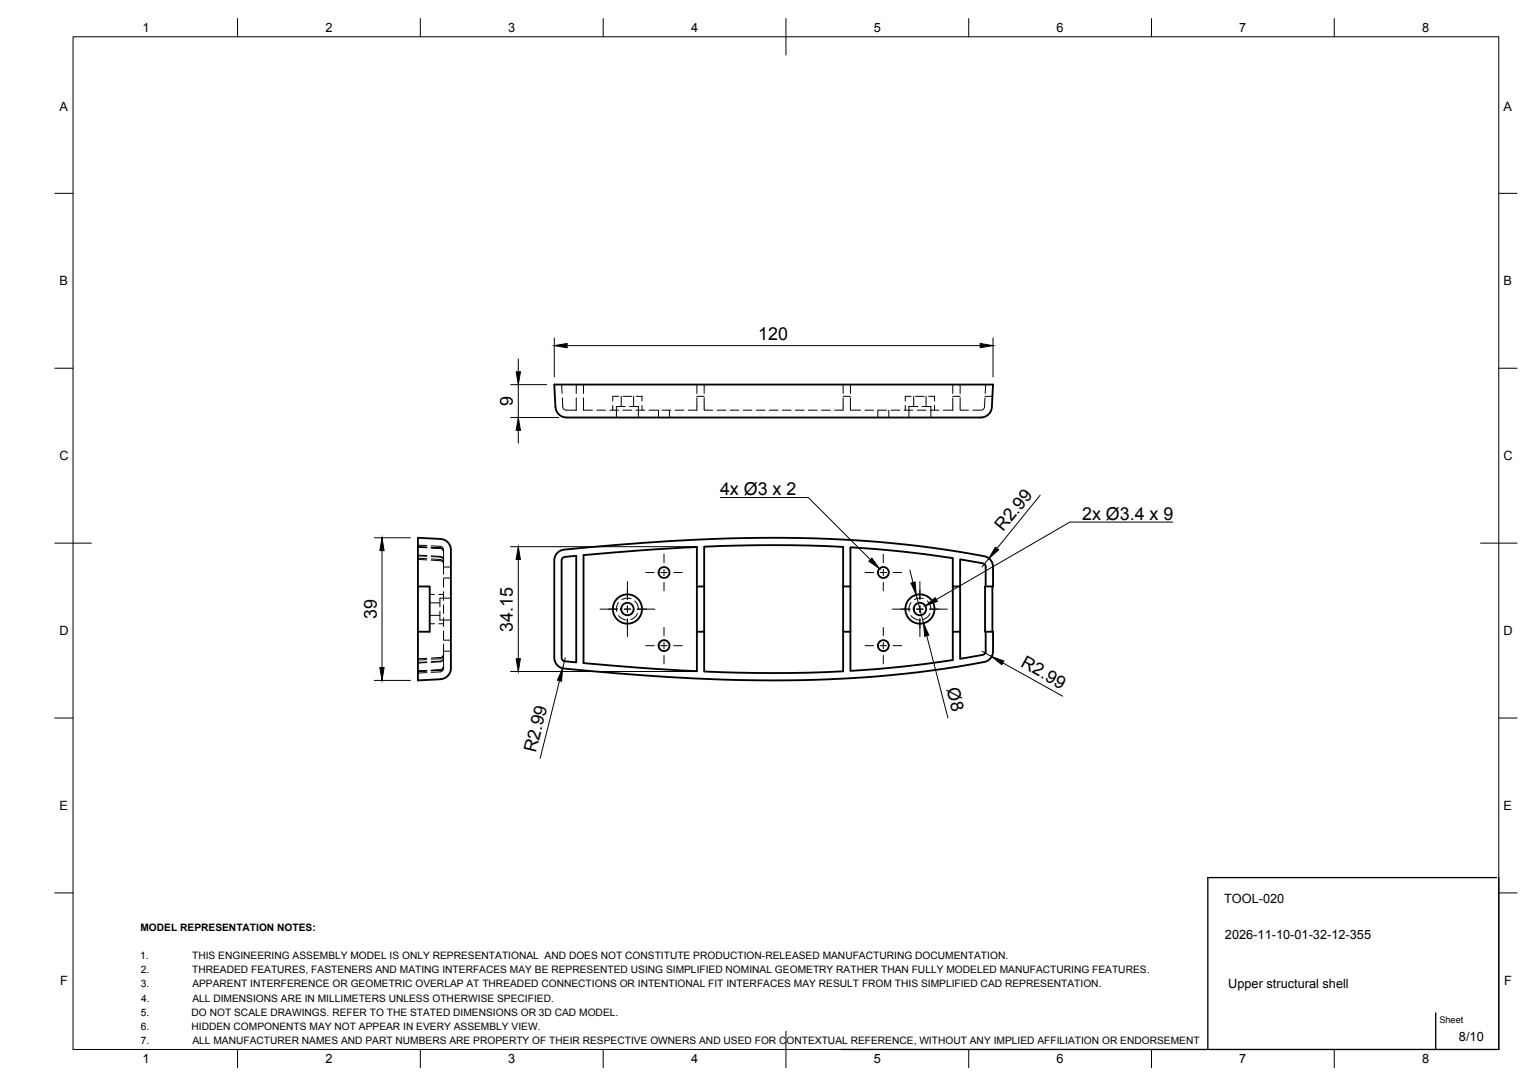
ISO-10303-21;
HEADER;
/* Generated by software containing ST-Developer
 * from STEP Tools, Inc. (www.steptools.com) 
 */

FILE_DESCRIPTION(
/* description */ (''),
/* implementation_level */ '2;1');

FILE_NAME(
/* name */ 'Upper structural shell.step',
/* time_stamp */ '2026-11-10T09:09:39-08:00',
/* author */ (''),
/* organization */ (''),
/* preprocessor_version */ 'ST-DEVELOPER v20.2',
/* originating_system */ 'Autodesk Translation Framework v15.17.0.0',
/* authorisation */ '');

FILE_SCHEMA (('AUTOMOTIVE_DESIGN { 1 0 10303 214 3 1 1 }'));
ENDSEC;

DATA;
#10=MECHANICAL_DESIGN_GEOMETRIC_PRESENTATION_REPRESENTATION('',(#558),#18353);
#75=SPHERICAL_SURFACE('',#6751,0.0999999999999999);
#76=SPHERICAL_SURFACE('',#6754,0.100000000000002);
#77=SPHERICAL_SURFACE('',#6758,0.0999999999999991);
#78=SPHERICAL_SURFACE('',#6762,0.1);
#79=SPHERICAL_SURFACE('',#6767,0.3);
#80=SPHERICAL_SURFACE('',#6771,0.300000000000002);
#81=SPHERICAL_SURFACE('',#6775,0.299999999999999);
#82=SPHERICAL_SURFACE('',#6780,0.3);
#91=B_SPLINE_SURFACE_WITH_KNOTS('',3,3,((#9570,#9571,#9572,#9573),(#9574,
#9575,#9576,#9577),(#9578,#9579,#9580,#9581),(#9582,#9583,#9584,#9585)),
 .UNSPECIFIED.,.F.,.F.,.F.,(4,4),(4,4),(0.0627625298587661,0.3242096015809),
(0.0118073085896899,0.685451490706028),.UNSPECIFIED.);
#92=B_SPLINE_SURFACE_WITH_KNOTS('',3,3,((#9590,#9591,#9592,#9593),(#9594,
#9595,#9596,#9597),(#9598,#9599,#9600,#9601),(#9602,#9603,#9604,#9605)),
 .UNSPECIFIED.,.F.,.F.,.F.,(4,4),(4,4),(0.0225360950145449,0.0483865590996774),
(0.0125659096559557,0.685650832343257),.UNSPECIFIED.);
#93=B_SPLINE_SURFACE_WITH_KNOTS('',3,3,((#9615,#9616,#9617,#9618),(#9619,
#9620,#9621,#9622),(#9623,#9624,#9625,#9626),(#9627,#9628,#9629,#9630),
(#9631,#9632,#9633,#9634)),.UNSPECIFIED.,.F.,.F.,.F.,(4,1,4),(4,4),(0.,
0.571428571428571,1.),(0.74118252158834,3.85438678954986),.UNSPECIFIED.);
#94=B_SPLINE_SURFACE_WITH_KNOTS('',3,3,((#9639,#9640,#9641,#9642),(#9643,
#9644,#9645,#9646),(#9647,#9648,#9649,#9650),(#9651,#9652,#9653,#9654),
(#9655,#9656,#9657,#9658)),.UNSPECIFIED.,.F.,.F.,.F.,(4,1,4),(4,4),(0.,
0.571428571428571,1.),(0.270878787657975,0.54981857912664),
 .UNSPECIFIED.);
#95=B_SPLINE_SURFACE_WITH_KNOTS('',3,3,((#9677,#9678,#9679,#9680),(#9681,
#9682,#9683,#9684),(#9685,#9686,#9687,#9688),(#9689,#9690,#9691,#9692),
(#9693,#9694,#9695,#9696)),.UNSPECIFIED.,.F.,.F.,.F.,(4,1,4),(4,4),(0.,
0.571428571428571,1.),(8.03948512627517,11.1526893942367),.UNSPECIFIED.);
#96=B_SPLINE_SURFACE_WITH_KNOTS('',3,3,((#9701,#9702,#9703,#9704),(#9705,
#9706,#9707,#9708),(#9709,#9710,#9711,#9712),(#9713,#9714,#9715,#9716)),
 .UNSPECIFIED.,.F.,.F.,.F.,(4,4),(4,4),(0.675790398419059,0.937237470141233),
(0.0118073085603101,0.685451490706029),.UNSPECIFIED.);
#97=B_SPLINE_SURFACE_WITH_KNOTS('',3,3,((#9717,#9718,#9719,#9720),(#9721,
#9722,#9723,#9724),(#9725,#9726,#9727,#9728),(#9729,#9730,#9731,#9732)),
 .UNSPECIFIED.,.F.,.F.,.F.,(4,4),(4,4),(0.951613440900322,0.977463904985455),
(0.0125659096559558,0.685650832343257),.UNSPECIFIED.);
#98=B_SPLINE_SURFACE_WITH_KNOTS('',3,3,((#9816,#9817,#9818,#9819),(#9820,
#9821,#9822,#9823),(#9824,#9825,#9826,#9827),(#9828,#9829,#9830,#9831)),
 .UNSPECIFIED.,.F.,.F.,.F.,(4,4),(4,4),(0.340089900275858,0.660082688299826),
(0.0116294244283504,0.684384408933581),.UNSPECIFIED.);
#99=B_SPLINE_SURFACE_WITH_KNOTS('',3,3,((#9836,#9837,#9838,#9839),(#9840,
#9841,#9842,#9843),(#9844,#9845,#9846,#9847),(#9848,#9849,#9850,#9851),
(#9852,#9853,#9854,#9855)),.UNSPECIFIED.,.F.,.F.,.F.,(4,1,4),(4,4),(0.,
0.571428571428571,1.),(4.04989375377528,7.85140214144331),.UNSPECIFIED.);
#100=B_SPLINE_SURFACE_WITH_KNOTS('',3,3,((#9865,#9866,#9867,#9868),(#9869,
#9870,#9871,#9872),(#9873,#9874,#9875,#9876),(#9877,#9878,#9879,#9880),
(#9881,#9882,#9883,#9884)),.UNSPECIFIED.,.F.,.F.,.F.,(4,1,4),(4,4),(0.,
0.571428571428571,1.),(4.0424697743818,7.84397816204974),.UNSPECIFIED.);
#101=B_SPLINE_SURFACE_WITH_KNOTS('',3,3,((#9889,#9890,#9891,#9892),(#9893,
#9894,#9895,#9896),(#9897,#9898,#9899,#9900),(#9901,#9902,#9903,#9904)),
 .UNSPECIFIED.,.F.,.F.,.F.,(4,4),(4,4),(0.339917311700174,0.659910099724142),
(0.0116294573698948,0.684384408933581),.UNSPECIFIED.);
#102=B_SPLINE_SURFACE_WITH_KNOTS('',3,3,((#9979,#9980,#9981,#9982),(#9983,
#9984,#9985,#9986),(#9987,#9988,#9989,#9990),(#9991,#9992,#9993,#9994)),
 .UNSPECIFIED.,.F.,.F.,.F.,(4,4),(4,4),(0.675996615945502,0.913173856075534),
(0.0118505108223707,0.686152089762332),.UNSPECIFIED.);
#103=B_SPLINE_SURFACE_WITH_KNOTS('',3,3,((#9999,#10000,#10001,#10002),(#10003,
#10004,#10005,#10006),(#10007,#10008,#10009,#10010),(#10011,#10012,#10013,
#10014),(#10015,#10016,#10017,#10018)),.UNSPECIFIED.,.F.,.F.,.F.,(4,1,4),
(4,4),(0.,0.571428571428571,1.),(8.0457708503995,10.8690635835914),
 .UNSPECIFIED.);
#104=B_SPLINE_SURFACE_WITH_KNOTS('',3,3,((#10028,#10029,#10030,#10031),
(#10032,#10033,#10034,#10035),(#10036,#10037,#10038,#10039),(#10040,#10041,
#10042,#10043),(#10044,#10045,#10046,#10047)),.UNSPECIFIED.,.F.,.F.,.F.,
(4,1,4),(4,4),(0.,0.571428571428571,1.),(1.02480833223363,3.8481010654256),
 .UNSPECIFIED.);
#105=B_SPLINE_SURFACE_WITH_KNOTS('',3,3,((#10052,#10053,#10054,#10055),
(#10056,#10057,#10058,#10059),(#10060,#10061,#10062,#10063),(#10064,#10065,
#10066,#10067)),.UNSPECIFIED.,.F.,.F.,.F.,(4,4),(4,4),(0.0868261439244655,
0.324003384054498),(0.0118505108223707,0.686152089762332),.UNSPECIFIED.);
#106=B_SPLINE_SURFACE_WITH_KNOTS('',3,3,((#10142,#10143,#10144,#10145),
(#10146,#10147,#10148,#10149),(#10150,#10151,#10152,#10153),(#10154,#10155,
#10156,#10157)),.UNSPECIFIED.,.F.,.F.,.F.,(4,4),(4,4),(0.927751606342899,
0.979699913047832),(0.0130895688562318,0.686930956013783),.UNSPECIFIED.);
#107=B_SPLINE_SURFACE_WITH_KNOTS('',3,3,((#10167,#10168,#10169,#10170),
(#10171,#10172,#10173,#10174),(#10175,#10176,#10177,#10178),(#10179,#10180,
#10181,#10182),(#10183,#10184,#10185,#10186)),.UNSPECIFIED.,.F.,.F.,.F.,
(4,1,4),(4,4),(0.,0.571428571428571,1.),(11.0550486447215,11.6488871259622),
 .UNSPECIFIED.);
#108=B_SPLINE_SURFACE_WITH_KNOTS('',3,3,((#10200,#10201,#10202,#10203),
(#10204,#10205,#10206,#10207),(#10208,#10209,#10210,#10211),(#10212,#10213,
#10214,#10215)),.UNSPECIFIED.,.F.,.F.,.F.,(4,4),(4,4),(0.0203000869521683,
0.0722483936571013),(0.0130895688562318,0.686930956013783),
 .UNSPECIFIED.);
#109=B_SPLINE_SURFACE_WITH_KNOTS('',3,3,((#10225,#10226,#10227,#10228),
(#10229,#10230,#10231,#10232),(#10233,#10234,#10235,#10236),(#10237,#10238,
#10239,#10240),(#10241,#10242,#10243,#10244)),.UNSPECIFIED.,.F.,.F.,.F.,
(4,1,4),(4,4),(0.,0.571428571428571,1.),(0.244984789862841,0.838823271103535),
 .UNSPECIFIED.);
#110=B_SPLINE_SURFACE_WITH_KNOTS('',3,3,((#10258,#10259,#10260,#10261),
(#10262,#10263,#10264,#10265),(#10266,#10267,#10268,#10269),(#10270,#10271,
#10272,#10273),(#10274,#10275,#10276,#10277)),.UNSPECIFIED.,.F.,.F.,.F.,
(4,1,4),(4,4),(0.,0.5,1.),(0.0108921325678979,0.619909717328002),
 .UNSPECIFIED.);
#111=B_SPLINE_SURFACE_WITH_KNOTS('',3,3,((#10284,#10285,#10286,#10287),
(#10288,#10289,#10290,#10291),(#10292,#10293,#10294,#10295),(#10296,#10297,
#10298,#10299),(#10300,#10301,#10302,#10303)),.UNSPECIFIED.,.F.,.F.,.F.,
(4,1,4),(4,4),(0.,0.571428571428571,1.),(0.00967450486392679,0.618764321025346),
 .UNSPECIFIED.);
#112=B_SPLINE_SURFACE_WITH_KNOTS('',3,3,((#10308,#10309,#10310,#10311),
(#10312,#10313,#10314,#10315),(#10316,#10317,#10318,#10319),(#10320,#10321,
#10322,#10323),(#10324,#10325,#10326,#10327)),.UNSPECIFIED.,.F.,.F.,.F.,
(4,1,4),(4,4),(0.,0.571428571428571,1.),(0.0097274579809394,0.618764321025346),
 .UNSPECIFIED.);
#113=B_SPLINE_SURFACE_WITH_KNOTS('',3,3,((#10332,#10333,#10334,#10335),
(#10336,#10337,#10338,#10339),(#10340,#10341,#10342,#10343),(#10344,#10345,
#10346,#10347),(#10348,#10349,#10350,#10351)),.UNSPECIFIED.,.F.,.F.,.F.,
(4,1,4),(4,4),(0.,0.571428571428571,1.),(11.3440533366984,11.6229931281671),
 .UNSPECIFIED.);
#114=B_SPLINE_SURFACE_WITH_KNOTS('',3,3,((#10352,#10353,#10354,#10355),
(#10356,#10357,#10358,#10359),(#10360,#10361,#10362,#10363),(#10364,#10365,
#10366,#10367),(#10368,#10369,#10370,#10371)),.UNSPECIFIED.,.F.,.F.,.F.,
(4,1,4),(4,4),(0.,0.5,1.),(0.0108402259132964,0.619909717328002),
 .UNSPECIFIED.);
#115=B_SPLINE_SURFACE_WITH_KNOTS('',3,3,((#10397,#10398,#10399,#10400),
(#10401,#10402,#10403,#10404),(#10405,#10406,#10407,#10408),(#10409,#10410,
#10411,#10412),(#10413,#10414,#10415,#10416)),.UNSPECIFIED.,.F.,.F.,.F.,
(4,1,4),(4,4),(0.,0.571428571428571,1.),(-0.00387706229521417,0.619909717328002),
 .UNSPECIFIED.);
#116=B_SPLINE_SURFACE_WITH_KNOTS('',3,3,((#10435,#10436,#10437,#10438,#10439,
#10440),(#10441,#10442,#10443,#10444,#10445,#10446),(#10447,#10448,#10449,
#10450,#10451,#10452),(#10453,#10454,#10455,#10456,#10457,#10458),(#10459,
#10460,#10461,#10462,#10463,#10464)),.UNSPECIFIED.,.F.,.F.,.F.,(4,1,4),
(4,1,1,4),(0.,0.571428571428571,1.),(0.270878787657975,5.14716807550265,
8.39802760073243,11.6488871259622),.UNSPECIFIED.);
#117=B_SPLINE_SURFACE_WITH_KNOTS('',3,3,((#10477,#10478,#10479,#10480),
(#10481,#10482,#10483,#10484),(#10485,#10486,#10487,#10488),(#10489,#10490,
#10491,#10492),(#10493,#10494,#10495,#10496)),.UNSPECIFIED.,.F.,.F.,.F.,
(4,1,4),(4,4),(0.,0.571428571428571,1.),(-0.00522825793187074,0.618764321025346),
 .UNSPECIFIED.);
#118=B_SPLINE_SURFACE_WITH_KNOTS('',3,3,((#10505,#10506,#10507,#10508),
(#10509,#10510,#10511,#10512),(#10513,#10514,#10515,#10516),(#10517,#10518,
#10519,#10520),(#10521,#10522,#10523,#10524)),.UNSPECIFIED.,.F.,.F.,.F.,
(4,1,4),(4,4),(0.,0.571428571428571,1.),(-0.00506942997988007,0.618764321025346),
 .UNSPECIFIED.);
#119=B_SPLINE_SURFACE_WITH_KNOTS('',3,3,((#10533,#10534,#10535,#10536,#10537),
(#10538,#10539,#10540,#10541,#10542),(#10543,#10544,#10545,#10546,#10547),
(#10548,#10549,#10550,#10551,#10552),(#10553,#10554,#10555,#10556,#10557)),
 .UNSPECIFIED.,.F.,.F.,.F.,(4,1,4),(4,1,4),(0.,0.571428571428571,1.),(0.244984789862841,
5.12127407770751,11.6229931281671),.UNSPECIFIED.);
#120=B_SPLINE_SURFACE_WITH_KNOTS('',3,3,((#10568,#10569,#10570,#10571),
(#10572,#10573,#10574,#10575),(#10576,#10577,#10578,#10579),(#10580,#10581,
#10582,#10583),(#10584,#10585,#10586,#10587)),.UNSPECIFIED.,.F.,.F.,.F.,
(4,1,4),(4,4),(0.,0.571428571428571,1.),(-0.00403278922781227,0.619909717328002),
 .UNSPECIFIED.);
#121=B_SPLINE_SURFACE_WITH_KNOTS('',3,3,((#10596,#10597,#10598,#10599),
(#10600,#10601,#10602,#10603),(#10604,#10605,#10606,#10607),(#10608,#10609,
#10610,#10611)),.UNSPECIFIED.,.F.,.F.,.F.,(4,4),(4,4),(0.0225340877622934,
0.979701609653785),(0.,0.686930956013783),.UNSPECIFIED.);
#122=B_SPLINE_SURFACE_WITH_KNOTS('',3,3,((#10614,#10615,#10616,#10617),
(#10618,#10619,#10620,#10621),(#10622,#10623,#10624,#10625),(#10626,#10627,
#10628,#10629)),.UNSPECIFIED.,.F.,.F.,.F.,(4,4),(4,4),(0.0202983903462145,
0.977465912237707),(0.,0.686930956013783),.UNSPECIFIED.);
#171=B_SPLINE_CURVE_WITH_KNOTS('',3,(#8842,#8843,#8844,#8845,#8846,#8847),
 .UNSPECIFIED.,.F.,.F.,(4,2,4),(-0.607240122656937,-0.303691721894415,-0.000634514333697656),
 .UNSPECIFIED.);
#172=B_SPLINE_CURVE_WITH_KNOTS('',3,(#8849,#8850,#8851,#8852,#8853,#8854,
#8855,#8856,#8857,#8858,#8859,#8860,#8861,#8862,#8863,#8864,#8865,#8866,
#8867,#8868,#8869,#8870,#8871,#8872,#8873,#8874,#8875,#8876),
 .UNSPECIFIED.,.F.,.F.,(4,3,3,3,3,3,3,3,3,4),(-0.152223584381152,-0.128403685910756,
-0.115058138924018,-0.0911105876986024,-0.0779275105489685,-0.0651650823668383,
-0.0413494676927402,-0.0389105926748606,-0.0151313403168948,0.),
 .UNSPECIFIED.);
#173=B_SPLINE_CURVE_WITH_KNOTS('',3,(#8880,#8881,#8882,#8883,#8884,#8885,
#8886,#8887,#8888,#8889,#8890,#8891,#8892,#8893,#8894,#8895,#8896,#8897,
#8898,#8899,#8900,#8901,#8902,#8903,#8904,#8905,#8906,#8907),
 .UNSPECIFIED.,.F.,.F.,(4,3,3,3,3,3,3,3,3,4),(-0.152249917238265,-0.128484865669312,
-0.115494642307313,-0.0916985948709881,-0.0870953287403626,-0.0787006597758974,
-0.0547717013112817,-0.0393956522318865,-0.0155460991587222,0.),
 .UNSPECIFIED.);
#174=B_SPLINE_CURVE_WITH_KNOTS('',3,(#8908,#8909,#8910,#8911,#8912,#8913),
 .UNSPECIFIED.,.F.,.F.,(4,2,4),(-0.606785315485727,-0.30369188913634,-0.000179692314978108),
 .UNSPECIFIED.);
#175=B_SPLINE_CURVE_WITH_KNOTS('',3,(#8918,#8919,#8920,#8921,#8922,#8923),
 .UNSPECIFIED.,.F.,.F.,(4,2,4),(-0.606332812995025,-0.303737653350621,-0.000161665236032726),
 .UNSPECIFIED.);
#176=B_SPLINE_CURVE_WITH_KNOTS('',3,(#8925,#8926,#8927,#8928,#8929,#8930,
#8931,#8932,#8933,#8934,#8935,#8936,#8937,#8938,#8939,#8940,#8941,#8942,
#8943,#8944,#8945,#8946,#8947,#8948,#8949,#8950,#8951,#8952),
 .UNSPECIFIED.,.F.,.F.,(4,3,3,3,3,3,3,3,3,4),(-0.152301160038588,-0.128555435257278,
-0.115184785848022,-0.0912639339035621,-0.0780773216554274,-0.065267350293706,
-0.0414723266145325,-0.0390252168402571,-0.0152374671294611,0.),
 .UNSPECIFIED.);
#177=B_SPLINE_CURVE_WITH_KNOTS('',3,(#8956,#8957,#8958,#8959,#8960,#8961,
#8962,#8963,#8964,#8965,#8966,#8967,#8968,#8969,#8970,#8971,#8972,#8973,
#8974,#8975,#8976,#8977,#8978,#8979,#8980,#8981,#8982,#8983),
 .UNSPECIFIED.,.F.,.F.,(4,3,3,3,3,3,3,3,3,4),(-0.152307894271445,-0.128535938708366,
-0.115295945509717,-0.0915234088298753,-0.0870575315710991,-0.0782740392368046,
-0.0543664511067997,-0.0391484926712317,-0.0153774171089249,0.),
 .UNSPECIFIED.);
#178=B_SPLINE_CURVE_WITH_KNOTS('',3,(#8985,#8986,#8987,#8988,#8989,#8990),
 .UNSPECIFIED.,.F.,.F.,(4,2,4),(-0.607315067615316,-0.303737782617996,-0.00114390098251854),
 .UNSPECIFIED.);
#179=B_SPLINE_CURVE_WITH_KNOTS('',3,(#8996,#8997,#8998,#8999,#9000,#9001),
 .UNSPECIFIED.,.F.,.F.,(4,2,4),(-0.606335618682527,-0.303964064424246,-0.000163142902895597),
 .UNSPECIFIED.);
#180=B_SPLINE_CURVE_WITH_KNOTS('',3,(#9003,#9004,#9005,#9006,#9007,#9008,
#9009,#9010,#9011,#9012,#9013,#9014,#9015,#9016,#9017,#9018,#9019,#9020,
#9021,#9022,#9023,#9024,#9025,#9026,#9027,#9028,#9029,#9030),
 .UNSPECIFIED.,.F.,.F.,(4,3,3,3,3,3,3,3,3,4),(-0.152324888062519,-0.128571266282871,
-0.115187819092559,-0.0912644922975459,-0.0780623053857969,-0.0652705430018984,
-0.0414736125245103,-0.0390138150290758,-0.015226502089553,0.),
 .UNSPECIFIED.);
#181=B_SPLINE_CURVE_WITH_KNOTS('',3,(#9034,#9035,#9036,#9037,#9038,#9039,
#9040,#9041,#9042,#9043,#9044,#9045,#9046,#9047,#9048,#9049,#9050,#9051,
#9052,#9053,#9054,#9055,#9056,#9057,#9058,#9059,#9060,#9061),
 .UNSPECIFIED.,.F.,.F.,(4,3,3,3,3,3,3,3,3,4),(-0.152333600285603,-0.128561769460285,
-0.115331525958272,-0.0915566852459163,-0.0870792380259527,-0.0783165909319309,
-0.0544069520497563,-0.0391732033593778,-0.0153939862842036,0.),
 .UNSPECIFIED.);
#182=B_SPLINE_CURVE_WITH_KNOTS('',3,(#9063,#9064,#9065,#9066,#9067,#9068),
 .UNSPECIFIED.,.F.,.F.,(4,2,4),(-0.607765665607205,-0.303964210965506,-0.00159316434717749),
 .UNSPECIFIED.);
#183=B_SPLINE_CURVE_WITH_KNOTS('',3,(#9074,#9075,#9076,#9077,#9078,#9079),
 .UNSPECIFIED.,.F.,.F.,(4,2,4),(-0.608113833554089,-0.304405910662044,-0.00120843896277512),
 .UNSPECIFIED.);
#184=B_SPLINE_CURVE_WITH_KNOTS('',3,(#9081,#9082,#9083,#9084,#9085,#9086,
#9087,#9088,#9089,#9090,#9091,#9092,#9093,#9094,#9095,#9096,#9097,#9098,
#9099,#9100,#9101,#9102,#9103,#9104,#9105,#9106,#9107,#9108),
 .UNSPECIFIED.,.F.,.F.,(4,3,3,3,3,3,3,3,3,4),(-0.152638346832965,-0.128647829044501,
-0.117000727359648,-0.0929750760194364,-0.0775532335837778,-0.065166230851578,
-0.0413072760700971,-0.0386249916896363,-0.0148681833632798,0.),
 .UNSPECIFIED.);
#185=B_SPLINE_CURVE_WITH_KNOTS('',3,(#9112,#9113,#9114,#9115,#9116,#9117,
#9118,#9119,#9120,#9121,#9122,#9123,#9124,#9125,#9126,#9127,#9128,#9129,
#9130,#9131,#9132,#9133,#9134,#9135,#9136,#9137,#9138,#9139),
 .UNSPECIFIED.,.F.,.F.,(4,3,3,3,3,3,3,3,3,4),(-0.152712908768378,-0.128963682254188,
-0.116304008925778,-0.092453135123643,-0.0875380734791113,-0.0797852913889514,
-0.0558105568475602,-0.0400274901149945,-0.0159798645019078,0.),
 .UNSPECIFIED.);
#186=B_SPLINE_CURVE_WITH_KNOTS('',3,(#9141,#9142,#9143,#9144,#9145,#9146),
 .UNSPECIFIED.,.F.,.F.,(4,2,4),(-0.607607610897069,-0.304406883675693,-0.000702187548907163),
 .UNSPECIFIED.);
#187=B_SPLINE_CURVE_WITH_KNOTS('',3,(#9152,#9153,#9154,#9155),
 .UNSPECIFIED.,.F.,.F.,(4,4),(0.0130288733793136,0.619909717328002),
 .UNSPECIFIED.);
#188=B_SPLINE_CURVE_WITH_KNOTS('',3,(#9159,#9160,#9161,#9162),
 .UNSPECIFIED.,.F.,.F.,(4,4),(-0.619909717328002,-0.0130288733793137),
 .UNSPECIFIED.);
#189=B_SPLINE_CURVE_WITH_KNOTS('',3,(#9165,#9166,#9167,#9168,#9169,#9170,
#9171),.UNSPECIFIED.,.F.,.F.,(4,3,4),(7.87274532319472,10.4298004347969,
10.9780233963721),.UNSPECIFIED.);
#190=B_SPLINE_CURVE_WITH_KNOTS('',3,(#9172,#9173,#9174,#9175,#9176,#9177,
#9178),.UNSPECIFIED.,.F.,.F.,(4,3,4),(0.511752108249611,2.84807862798167,
3.61537599721027),.UNSPECIFIED.);
#191=B_SPLINE_CURVE_WITH_KNOTS('',3,(#9181,#9182,#9183,#9184,#9185,#9186,
#9187),.UNSPECIFIED.,.F.,.F.,(4,3,4),(3.81523717927831,5.72635044542746,
7.61820606472736),.UNSPECIFIED.);
#192=B_SPLINE_CURVE_WITH_KNOTS('',3,(#9190,#9191,#9192,#9193),
 .UNSPECIFIED.,.F.,.F.,(4,4),(7.8195516254834,10.6519234170402),
 .UNSPECIFIED.);
#193=B_SPLINE_CURVE_WITH_KNOTS('',3,(#9197,#9198,#9199,#9200),
 .UNSPECIFIED.,.F.,.F.,(4,4),(10.8550709503701,11.4839159448819),
 .UNSPECIFIED.);
#194=B_SPLINE_CURVE_WITH_KNOTS('',3,(#9201,#9202,#9203,#9204,#9205,#9206,
#9207,#9208,#9209,#9210,#9211,#9212,#9213,#9214,#9215,#9216,#9217,#9218,
#9219,#9220,#9221,#9222,#9223,#9224,#9225,#9226,#9227,#9228),
 .UNSPECIFIED.,.F.,.F.,(4,3,3,3,3,3,3,3,3,4),(0.,0.023800266251022,0.0390470051780055,
0.062864594207143,0.0692752090304052,0.0780196763370091,0.101808338076191,
0.108235461704482,0.131970324379069,0.138468980573541),.UNSPECIFIED.);
#195=B_SPLINE_CURVE_WITH_KNOTS('',3,(#9232,#9233,#9234,#9235,#9236,#9237,
#9238,#9239,#9240,#9241,#9242,#9243,#9244,#9245,#9246,#9247,#9248,#9249,
#9250,#9251,#9252,#9253,#9254,#9255,#9256,#9257,#9258,#9259,#9260,#9261,
#9262),.UNSPECIFIED.,.F.,.F.,(4,3,3,3,3,3,3,3,3,3,4),(0.,0.0536158767337707,
0.107707970980176,0.117140678528723,0.171373940961503,0.178118425384842,
0.234058785038521,0.2884659822146,0.324708667187819,0.378759781373182,0.415412568437851),
 .UNSPECIFIED.);
#196=B_SPLINE_CURVE_WITH_KNOTS('',3,(#9264,#9265,#9266,#9267),
 .UNSPECIFIED.,.F.,.F.,(4,4),(0.0202983903462145,0.977465912237707),
 .UNSPECIFIED.);
#197=B_SPLINE_CURVE_WITH_KNOTS('',3,(#9269,#9270,#9271,#9272,#9273,#9274,
#9275,#9276,#9277,#9278,#9279,#9280,#9281,#9282,#9283,#9284,#9285,#9286,
#9287,#9288,#9289,#9290,#9291,#9292,#9293,#9294,#9295,#9296,#9297,#9298,
#9299),.UNSPECIFIED.,.F.,.F.,(4,3,3,3,3,3,3,3,3,3,4),(0.,0.053547205187505,
0.107728964525782,0.117299670245694,0.171524652009909,0.189842726242433,
0.234296321023441,0.288773621215207,0.338477936388461,0.392564001789548,
0.442713223041249),.UNSPECIFIED.);
#198=B_SPLINE_CURVE_WITH_KNOTS('',3,(#9303,#9304,#9305,#9306,#9307,#9308,
#9309,#9310,#9311,#9312,#9313,#9314,#9315,#9316,#9317,#9318,#9319,#9320,
#9321,#9322,#9323,#9324,#9325,#9326,#9327,#9328,#9329,#9330,#9331,#9332,
#9333),.UNSPECIFIED.,.F.,.F.,(4,3,3,3,3,3,3,3,3,3,4),(0.,0.0535312152416108,
0.107707123412492,0.117215931328448,0.171445047002381,0.189808362521926,
0.234165405003858,0.288639615809812,0.338404447092272,0.392504428396833,
0.442708851597914),.UNSPECIFIED.);
#199=B_SPLINE_CURVE_WITH_KNOTS('',3,(#9335,#9336,#9337,#9338),
 .UNSPECIFIED.,.F.,.F.,(4,4),(0.0225340877622936,0.979701609653785),
 .UNSPECIFIED.);
#200=B_SPLINE_CURVE_WITH_KNOTS('',3,(#9340,#9341,#9342,#9343,#9344,#9345,
#9346,#9347,#9348,#9349,#9350,#9351,#9352,#9353,#9354,#9355,#9356,#9357,
#9358,#9359,#9360,#9361,#9362,#9363,#9364,#9365,#9366,#9367,#9368,#9369,
#9370),.UNSPECIFIED.,.F.,.F.,(4,3,3,3,3,3,3,3,3,3,4),(0.,0.0536458552170769,
0.107744721567334,0.117297895480617,0.171522683869793,0.178177673384308,
0.23429412186666,0.288702228477357,0.324838815929715,0.378862861687027,
0.415420074045746),.UNSPECIFIED.);
#201=B_SPLINE_CURVE_WITH_KNOTS('',3,(#9373,#9374,#9375,#9376,#9377,#9378,
#9379,#9380,#9381,#9382,#9383,#9384,#9385,#9386,#9387,#9388,#9389,#9390,
#9391,#9392,#9393,#9394,#9395,#9396,#9397,#9398,#9399,#9400),
 .UNSPECIFIED.,.F.,.F.,(4,3,3,3,3,3,3,3,3,4),(0.,0.0238098951475563,0.0390995920428052,
0.0629117710415135,0.0692953339558167,0.0780985718814299,0.101889748471939,
0.108278926258091,0.132003149848588,0.138471484390145),.UNSPECIFIED.);
#202=B_SPLINE_CURVE_WITH_KNOTS('',3,(#9402,#9403,#9404,#9405),
 .UNSPECIFIED.,.F.,.F.,(4,4),(2.05597917304345E-5,0.629200412657851),
 .UNSPECIFIED.);
#203=B_SPLINE_CURVE_WITH_KNOTS('',3,(#9408,#9409,#9410,#9411),
 .UNSPECIFIED.,.F.,.F.,(4,4),(0.832456091119126,3.6663340257767),
 .UNSPECIFIED.);
#204=B_SPLINE_CURVE_WITH_KNOTS('',3,(#9414,#9415,#9416,#9417,#9418,#9419,
#9420),.UNSPECIFIED.,.F.,.F.,(4,3,4),(3.86778652923942,5.76006783397632,
7.67277763234621),.UNSPECIFIED.);
#205=B_SPLINE_CURVE_WITH_KNOTS('',3,(#9424,#9425,#9426,#9427),
 .UNSPECIFIED.,.F.,.F.,(4,4),(11.1789026308149,11.490024089745),
 .UNSPECIFIED.);
#206=B_SPLINE_CURVE_WITH_KNOTS('',3,(#9429,#9430,#9431,#9432,#9433,#9434,
#9435,#9436,#9437,#9438,#9439,#9440,#9441,#9442,#9443,#9444,#9445,#9446,
#9447,#9448,#9449,#9450,#9451,#9452,#9453),.UNSPECIFIED.,.F.,.F.,(4,3,3,
3,3,3,3,3,4),(0.,0.0238050540413609,0.0390723036702896,0.0632692088215501,
0.0780555758269344,0.101951849921082,0.112801451778717,0.136536488207902,
0.147568670144067),.UNSPECIFIED.);
#207=B_SPLINE_CURVE_WITH_KNOTS('',3,(#9457,#9458,#9459,#9460,#9461,#9462,
#9463,#9464,#9465,#9466,#9467,#9468,#9469,#9470,#9471,#9472,#9473,#9474,
#9475,#9476,#9477,#9478,#9479,#9480,#9481),.UNSPECIFIED.,.F.,.F.,(4,3,3,
3,3,3,3,3,4),(0.,0.0238098889950854,0.0391003179068551,0.0632803937136523,
0.0780994777107358,0.101997157448698,0.112825962756833,0.136555142506291,
0.147570127973408),.UNSPECIFIED.);
#208=B_SPLINE_CURVE_WITH_KNOTS('',3,(#9483,#9484,#9485,#9486),
 .UNSPECIFIED.,.F.,.F.,(4,4),(2.41556456535008E-5,0.310979882704647),
 .UNSPECIFIED.);
#209=B_SPLINE_CURVE_WITH_KNOTS('',3,(#9498,#9499,#9500,#9501,#9502,#9503),
 .UNSPECIFIED.,.F.,.F.,(4,2,4),(-0.606744425054929,-0.30369469419025,-0.000104868936493974),
 .UNSPECIFIED.);
#210=B_SPLINE_CURVE_WITH_KNOTS('',3,(#9505,#9506,#9507,#9508,#9509,#9510),
 .UNSPECIFIED.,.F.,.F.,(4,2,4),(-0.60732337425873,-0.303694522808999,-0.000683832228057069),
 .UNSPECIFIED.);
#211=B_SPLINE_CURVE_WITH_KNOTS('',3,(#9512,#9513,#9514,#9515,#9516,#9517,
#9518,#9519,#9520,#9521,#9522,#9523,#9524,#9525,#9526,#9527,#9528,#9529,
#9530,#9531,#9532,#9533,#9534,#9535,#9536,#9537,#9538,#9539),
 .UNSPECIFIED.,.F.,.F.,(4,3,3,3,3,3,3,3,3,4),(-0.152213081758773,-0.128388856548194,
-0.115047734630008,-0.0910986092737131,-0.0779187269986961,-0.0651565114518209,
-0.0413397067626705,-0.0389038209724845,-0.0151251319644201,0.),
 .UNSPECIFIED.);
#212=B_SPLINE_CURVE_WITH_KNOTS('',3,(#9542,#9543,#9544,#9545,#9546,#9547,
#9548,#9549,#9550,#9551,#9552,#9553,#9554,#9555,#9556,#9557,#9558,#9559,
#9560,#9561,#9562,#9563,#9564,#9565,#9566,#9567,#9568,#9569),
 .UNSPECIFIED.,.F.,.F.,(4,3,3,3,3,3,3,3,3,4),(-0.152240567100014,-0.128476012965191,
-0.115503482174674,-0.0917060839439778,-0.0870941983819305,-0.0787260045726768,
-0.0547958477503903,-0.0394103419198022,-0.0155561788900784,0.),
 .UNSPECIFIED.);
#213=B_SPLINE_CURVE_WITH_KNOTS('',3,(#9586,#9587,#9588,#9589),
 .UNSPECIFIED.,.F.,.F.,(4,4),(-3.85438678954986,-0.750511952447855),
 .UNSPECIFIED.);
#214=B_SPLINE_CURVE_WITH_KNOTS('',3,(#9607,#9608,#9609,#9610),
 .UNSPECIFIED.,.F.,.F.,(4,4),(-0.54981857912664,-0.270878787657975),
 .UNSPECIFIED.);
#215=B_SPLINE_CURVE_WITH_KNOTS('',3,(#9611,#9612,#9613,#9614),
 .UNSPECIFIED.,.F.,.F.,(4,4),(-0.618764321025346,-0.0114172178585034),
 .UNSPECIFIED.);
#216=B_SPLINE_CURVE_WITH_KNOTS('',3,(#9635,#9636,#9637,#9638),
 .UNSPECIFIED.,.F.,.F.,(4,4),(0.74118252158834,3.84969085360113),
 .UNSPECIFIED.);
#217=B_SPLINE_CURVE_WITH_KNOTS('',3,(#9660,#9661,#9662,#9663),
 .UNSPECIFIED.,.F.,.F.,(4,4),(0.270878787657975,0.540284107299618),
 .UNSPECIFIED.);
#218=B_SPLINE_CURVE_WITH_KNOTS('',3,(#9666,#9667,#9668,#9669),
 .UNSPECIFIED.,.F.,.F.,(4,4),(8.04418106222393,11.1526893942367),
 .UNSPECIFIED.);
#219=B_SPLINE_CURVE_WITH_KNOTS('',3,(#9672,#9673,#9674,#9675),
 .UNSPECIFIED.,.F.,.F.,(4,4),(11.3535878085254,11.6229931281671),
 .UNSPECIFIED.);
#220=B_SPLINE_CURVE_WITH_KNOTS('',3,(#9697,#9698,#9699,#9700),
 .UNSPECIFIED.,.F.,.F.,(4,4),(-11.1433599633772,-8.03948512627517),
 .UNSPECIFIED.);
#221=B_SPLINE_CURVE_WITH_KNOTS('',3,(#9734,#9735,#9736,#9737),
 .UNSPECIFIED.,.F.,.F.,(4,4),(0.0114172178585033,0.618764321025346),
 .UNSPECIFIED.);
#222=B_SPLINE_CURVE_WITH_KNOTS('',3,(#9738,#9739,#9740,#9741),
 .UNSPECIFIED.,.F.,.F.,(4,4),(-11.6229931281671,-11.3440533366984),
 .UNSPECIFIED.);
#223=B_SPLINE_CURVE_WITH_KNOTS('',3,(#9744,#9745,#9746,#9747,#9748,#9749),
 .UNSPECIFIED.,.F.,.F.,(4,2,4),(-0.606286853269513,-0.303735636734938,-0.000134370544016882),
 .UNSPECIFIED.);
#224=B_SPLINE_CURVE_WITH_KNOTS('',3,(#9751,#9752,#9753,#9754,#9755,#9756,
#9757,#9758,#9759,#9760,#9761,#9762,#9763,#9764,#9765,#9766,#9767,#9768,
#9769,#9770,#9771,#9772,#9773,#9774,#9775,#9776,#9777,#9778),
 .UNSPECIFIED.,.F.,.F.,(4,3,3,3,3,3,3,3,3,4),(-0.152301724526365,-0.128559761662057,
-0.115189905045126,-0.0912708316251271,-0.0780855696141105,-0.0652713768517459,
-0.0414777101816728,-0.0390314967756457,-0.015242903619151,0.),
 .UNSPECIFIED.);
#225=B_SPLINE_CURVE_WITH_KNOTS('',3,(#9782,#9783,#9784,#9785,#9786,#9787,
#9788,#9789,#9790,#9791,#9792,#9793,#9794,#9795,#9796,#9797,#9798,#9799,
#9800,#9801,#9802,#9803,#9804,#9805,#9806,#9807,#9808,#9809),
 .UNSPECIFIED.,.F.,.F.,(4,3,3,3,3,3,3,3,3,4),(-0.1523073815286,-0.1285346644938,
-0.115283264026726,-0.0915123087981378,-0.0870533687950649,-0.0782507800682277,
-0.0543447803816484,-0.0391350231834537,-0.0153679399182895,0.),
 .UNSPECIFIED.);
#226=B_SPLINE_CURVE_WITH_KNOTS('',3,(#9810,#9811,#9812,#9813,#9814,#9815),
 .UNSPECIFIED.,.F.,.F.,(4,2,4),(-0.607338074051965,-0.303735662161239,-0.00118557149519966),
 .UNSPECIFIED.);
#227=B_SPLINE_CURVE_WITH_KNOTS('',3,(#9832,#9833,#9834,#9835),
 .UNSPECIFIED.,.F.,.F.,(4,4),(-7.8460657686783,-4.05419673417835),
 .UNSPECIFIED.);
#228=B_SPLINE_CURVE_WITH_KNOTS('',3,(#9856,#9857,#9858,#9859),
 .UNSPECIFIED.,.F.,.F.,(4,4),(4.04989375377528,7.85140214144331),
 .UNSPECIFIED.);
#229=B_SPLINE_CURVE_WITH_KNOTS('',3,(#9861,#9862,#9863,#9864),
 .UNSPECIFIED.,.F.,.F.,(4,4),(4.0424697743818,7.84397816204974),
 .UNSPECIFIED.);
#230=B_SPLINE_CURVE_WITH_KNOTS('',3,(#9885,#9886,#9887,#9888),
 .UNSPECIFIED.,.F.,.F.,(4,4),(-7.83967518164668,-4.0478061471468),
 .UNSPECIFIED.);
#231=B_SPLINE_CURVE_WITH_KNOTS('',3,(#9907,#9908,#9909,#9910,#9911,#9912),
 .UNSPECIFIED.,.F.,.F.,(4,2,4),(-0.606398914035431,-0.303967092551845,-0.000200694235479137),
 .UNSPECIFIED.);
#232=B_SPLINE_CURVE_WITH_KNOTS('',3,(#9914,#9915,#9916,#9917,#9918,#9919,
#9920,#9921,#9922,#9923,#9924,#9925,#9926,#9927,#9928,#9929,#9930,#9931,
#9932,#9933,#9934,#9935,#9936,#9937,#9938,#9939,#9940,#9941),
 .UNSPECIFIED.,.F.,.F.,(4,3,3,3,3,3,3,3,3,4),(-0.15233244131821,-0.128569871170003,
-0.115181988990177,-0.0912564475476021,-0.0780459432968613,-0.0652662335163151,
-0.0414674738832469,-0.0390013640446512,-0.0152139229936509,0.),
 .UNSPECIFIED.);
#233=B_SPLINE_CURVE_WITH_KNOTS('',3,(#9945,#9946,#9947,#9948,#9949,#9950,
#9951,#9952,#9953,#9954,#9955,#9956,#9957,#9958,#9959,#9960,#9961,#9962,
#9963,#9964,#9965,#9966,#9967,#9968,#9969,#9970,#9971,#9972),
 .UNSPECIFIED.,.F.,.F.,(4,3,3,3,3,3,3,3,3,4),(-0.152343297533924,-0.128571042154168,
-0.115361098257144,-0.0915841820623439,-0.0870924557961151,-0.0783628838319633,
-0.0544516462338148,-0.0392000432438046,-0.0154115240971992,0.),
 .UNSPECIFIED.);
#234=B_SPLINE_CURVE_WITH_KNOTS('',3,(#9973,#9974,#9975,#9976,#9977,#9978),
 .UNSPECIFIED.,.F.,.F.,(4,2,4),(-0.607734321217702,-0.303967174049374,-0.00153607519677973),
 .UNSPECIFIED.);
#235=B_SPLINE_CURVE_WITH_KNOTS('',3,(#9995,#9996,#9997,#9998),
 .UNSPECIFIED.,.F.,.F.,(4,4),(-10.8531956503852,-8.0457708503995),
 .UNSPECIFIED.);
#236=B_SPLINE_CURVE_WITH_KNOTS('',3,(#10019,#10020,#10021,#10022),
 .UNSPECIFIED.,.F.,.F.,(4,4),(8.05172912332209,10.8690635835914),
 .UNSPECIFIED.);
#237=B_SPLINE_CURVE_WITH_KNOTS('',3,(#10024,#10025,#10026,#10027),
 .UNSPECIFIED.,.F.,.F.,(4,4),(1.02480833223363,3.84214279250303),
 .UNSPECIFIED.);
#238=B_SPLINE_CURVE_WITH_KNOTS('',3,(#10048,#10049,#10050,#10051),
 .UNSPECIFIED.,.F.,.F.,(4,4),(-3.8481010654256,-1.04067626543981),
 .UNSPECIFIED.);
#239=B_SPLINE_CURVE_WITH_KNOTS('',3,(#10070,#10071,#10072,#10073,#10074,
#10075),.UNSPECIFIED.,.F.,.F.,(4,2,4),(-0.608301643694891,-0.304416323412316,
-0.0013178649037765),.UNSPECIFIED.);
#240=B_SPLINE_CURVE_WITH_KNOTS('',3,(#10077,#10078,#10079,#10080,#10081,
#10082,#10083,#10084,#10085,#10086,#10087,#10088,#10089,#10090,#10091,#10092,
#10093,#10094,#10095,#10096,#10097,#10098,#10099,#10100,#10101,#10102,#10103,
#10104),.UNSPECIFIED.,.F.,.F.,(4,3,3,3,3,3,3,3,3,4),(-0.152679905805259,
-0.128657903528546,-0.116982385578132,-0.0929502017086943,-0.0774957796939621,
-0.0651567901405441,-0.0412920018136918,-0.0385809476656748,-0.0148252868187304,
0.),.UNSPECIFIED.);
#241=B_SPLINE_CURVE_WITH_KNOTS('',3,(#10108,#10109,#10110,#10111,#10112,
#10113,#10114,#10115,#10116,#10117,#10118,#10119,#10120,#10121,#10122,#10123,
#10124,#10125,#10126,#10127,#10128,#10129,#10130,#10131,#10132,#10133,#10134,
#10135),.UNSPECIFIED.,.F.,.F.,(4,3,3,3,3,3,3,3,3,4),(-0.152762160496458,
-0.129013039804674,-0.116418683706179,-0.0925605502531877,-0.0875939536119484,
-0.0799546107253736,-0.055976748465099,-0.0401263304884301,-0.0160466564276224,
0.),.UNSPECIFIED.);
#242=B_SPLINE_CURVE_WITH_KNOTS('',3,(#10136,#10137,#10138,#10139,#10140,
#10141),.UNSPECIFIED.,.F.,.F.,(4,2,4),(-0.607519387555057,-0.304417308507995,
-0.000535579674449116),.UNSPECIFIED.);
#243=B_SPLINE_CURVE_WITH_KNOTS('',3,(#10159,#10160,#10161,#10162),
 .UNSPECIFIED.,.F.,.F.,(4,4),(0.012184405392802,0.619909717328002),
 .UNSPECIFIED.);
#244=B_SPLINE_CURVE_WITH_KNOTS('',3,(#10163,#10164,#10165,#10166),
 .UNSPECIFIED.,.F.,.F.,(4,4),(-11.6488871259622,-11.0550486447215),
 .UNSPECIFIED.);
#245=B_SPLINE_CURVE_WITH_KNOTS('',3,(#10189,#10190,#10191,#10192),
 .UNSPECIFIED.,.F.,.F.,(4,4),(11.0717103908866,11.6488871259622),
 .UNSPECIFIED.);
#246=B_SPLINE_CURVE_WITH_KNOTS('',3,(#10196,#10197,#10198,#10199),
 .UNSPECIFIED.,.F.,.F.,(4,4),(0.244984789862841,0.822161524938444),
 .UNSPECIFIED.);
#247=B_SPLINE_CURVE_WITH_KNOTS('',3,(#10217,#10218,#10219,#10220),
 .UNSPECIFIED.,.F.,.F.,(4,4),(-0.838823271103535,-0.244984789862841),
 .UNSPECIFIED.);
#248=B_SPLINE_CURVE_WITH_KNOTS('',3,(#10221,#10222,#10223,#10224),
 .UNSPECIFIED.,.F.,.F.,(4,4),(-0.619909717328002,-0.0121844053928019),
 .UNSPECIFIED.);
#249=B_SPLINE_CURVE_WITH_KNOTS('',3,(#10304,#10305,#10306,#10307),
 .UNSPECIFIED.,.F.,.F.,(4,4),(0.011877999214525,0.618764321025346),
 .UNSPECIFIED.);
#250=B_SPLINE_CURVE_WITH_KNOTS('',3,(#10328,#10329,#10330,#10331),
 .UNSPECIFIED.,.F.,.F.,(4,4),(-0.618764321025346,-0.0118779992145249),
 .UNSPECIFIED.);
#251=B_SPLINE_CURVE_WITH_KNOTS('',3,(#10417,#10418,#10419,#10420),
 .UNSPECIFIED.,.F.,.F.,(4,4),(-1.34441069388203E-17,0.619909717328002),
 .UNSPECIFIED.);
#252=B_SPLINE_CURVE_WITH_KNOTS('',3,(#10421,#10422,#10423,#10424),
 .UNSPECIFIED.,.F.,.F.,(4,4),(-0.619909717328002,-0.00253319281730041),
 .UNSPECIFIED.);
#253=B_SPLINE_CURVE_WITH_KNOTS('',3,(#10465,#10466,#10467,#10468,#10469,
#10470),.UNSPECIFIED.,.F.,.F.,(4,1,1,4),(-11.6488871259622,-8.39802760073243,
-5.14716807550265,-0.270878787657975),.UNSPECIFIED.);
#254=B_SPLINE_CURVE_WITH_KNOTS('',3,(#10471,#10472,#10473,#10474,#10475,
#10476),.UNSPECIFIED.,.F.,.F.,(4,1,1,4),(0.270878787657975,5.14716807550265,
8.39802760073243,11.6488871259622),.UNSPECIFIED.);
#255=B_SPLINE_CURVE_WITH_KNOTS('',3,(#10497,#10498,#10499,#10500),
 .UNSPECIFIED.,.F.,.F.,(4,4),(0.0013822243147816,0.618764321025346),
 .UNSPECIFIED.);
#256=B_SPLINE_CURVE_WITH_KNOTS('',3,(#10501,#10502,#10503,#10504),
 .UNSPECIFIED.,.F.,.F.,(4,4),(-0.618764321025346,8.06646416329215E-17),
 .UNSPECIFIED.);
#257=B_SPLINE_CURVE_WITH_KNOTS('',3,(#10525,#10526,#10527,#10528),
 .UNSPECIFIED.,.F.,.F.,(4,4),(-9.36750677027476E-17,0.618764321025346),
 .UNSPECIFIED.);
#258=B_SPLINE_CURVE_WITH_KNOTS('',3,(#10529,#10530,#10531,#10532),
 .UNSPECIFIED.,.F.,.F.,(4,4),(-0.618764321025346,-0.00138222431478148),
 .UNSPECIFIED.);
#259=B_SPLINE_CURVE_WITH_KNOTS('',3,(#10558,#10559,#10560,#10561,#10562),
 .UNSPECIFIED.,.F.,.F.,(4,1,4),(-11.6229931281671,-5.12127407770751,-0.244984789862841),
 .UNSPECIFIED.);
#260=B_SPLINE_CURVE_WITH_KNOTS('',3,(#10563,#10564,#10565,#10566,#10567),
 .UNSPECIFIED.,.F.,.F.,(4,1,4),(0.244984789862841,5.12127407770751,11.6229931281671),
 .UNSPECIFIED.);
#261=B_SPLINE_CURVE_WITH_KNOTS('',3,(#10588,#10589,#10590,#10591),
 .UNSPECIFIED.,.F.,.F.,(4,4),(0.00253319281730024,0.619909717328002),
 .UNSPECIFIED.);
#262=B_SPLINE_CURVE_WITH_KNOTS('',3,(#10592,#10593,#10594,#10595),
 .UNSPECIFIED.,.F.,.F.,(4,4),(-0.619909717328002,-2.51534904016637E-17),
 .UNSPECIFIED.);
#540=SHAPE_REPRESENTATION_RELATIONSHIP('SRR','None',#18401,#549);
#549=ADVANCED_BREP_SHAPE_REPRESENTATION('',(#567),#18347);
#558=STYLED_ITEM('',(#18459),#567);
#567=MANIFOLD_SOLID_BREP('Body1',#6489);
#586=FACE_BOUND('',#1219,.T.);
#587=FACE_BOUND('',#1222,.T.);
#588=FACE_BOUND('',#1233,.T.);
#589=FACE_BOUND('',#1235,.T.);
#590=FACE_BOUND('',#1247,.T.);
#591=FACE_BOUND('',#1256,.T.);
#592=FACE_BOUND('',#1257,.T.);
#593=FACE_BOUND('',#1258,.T.);
#594=FACE_BOUND('',#1273,.T.);
#595=FACE_BOUND('',#1274,.T.);
#596=FACE_BOUND('',#1275,.T.);
#597=FACE_BOUND('',#1311,.T.);
#598=FACE_BOUND('',#1312,.T.);
#599=FACE_BOUND('',#1313,.T.);
#600=FACE_BOUND('',#1314,.T.);
#601=FACE_BOUND('',#1315,.T.);
#602=FACE_BOUND('',#1316,.T.);
#668=PLANE('',#6702);
#669=PLANE('',#6707);
#670=PLANE('',#6713);
#671=PLANE('',#6714);
#672=PLANE('',#6715);
#673=PLANE('',#6716);
#674=PLANE('',#6717);
#675=PLANE('',#6718);
#676=PLANE('',#6719);
#677=PLANE('',#6720);
#678=PLANE('',#6722);
#679=PLANE('',#6724);
#680=PLANE('',#6725);
#681=PLANE('',#6726);
#682=PLANE('',#6727);
#683=PLANE('',#6728);
#684=PLANE('',#6729);
#685=PLANE('',#6730);
#686=PLANE('',#6731);
#687=PLANE('',#6732);
#688=PLANE('',#6733);
#689=PLANE('',#6734);
#690=PLANE('',#6739);
#691=PLANE('',#6741);
#692=PLANE('',#6742);
#693=PLANE('',#6743);
#694=PLANE('',#6744);
#695=PLANE('',#6745);
#696=PLANE('',#6746);
#697=PLANE('',#6747);
#698=PLANE('',#6749);
#699=PLANE('',#6766);
#700=PLANE('',#6785);
#701=PLANE('',#6786);
#702=PLANE('',#6787);
#829=FACE_OUTER_BOUND('',#1213,.T.);
#830=FACE_OUTER_BOUND('',#1214,.T.);
#831=FACE_OUTER_BOUND('',#1215,.T.);
#832=FACE_OUTER_BOUND('',#1216,.T.);
#833=FACE_OUTER_BOUND('',#1217,.T.);
#834=FACE_OUTER_BOUND('',#1218,.T.);
#835=FACE_OUTER_BOUND('',#1220,.T.);
#836=FACE_OUTER_BOUND('',#1221,.T.);
#837=FACE_OUTER_BOUND('',#1223,.T.);
#838=FACE_OUTER_BOUND('',#1224,.T.);
#839=FACE_OUTER_BOUND('',#1225,.T.);
#840=FACE_OUTER_BOUND('',#1226,.T.);
#841=FACE_OUTER_BOUND('',#1227,.T.);
#842=FACE_OUTER_BOUND('',#1228,.T.);
#843=FACE_OUTER_BOUND('',#1229,.T.);
#844=FACE_OUTER_BOUND('',#1230,.T.);
#845=FACE_OUTER_BOUND('',#1231,.T.);
#846=FACE_OUTER_BOUND('',#1232,.T.);
#847=FACE_OUTER_BOUND('',#1234,.T.);
#848=FACE_OUTER_BOUND('',#1236,.T.);
#849=FACE_OUTER_BOUND('',#1237,.T.);
#850=FACE_OUTER_BOUND('',#1238,.T.);
#851=FACE_OUTER_BOUND('',#1239,.T.);
#852=FACE_OUTER_BOUND('',#1240,.T.);
#853=FACE_OUTER_BOUND('',#1241,.T.);
#854=FACE_OUTER_BOUND('',#1242,.T.);
#855=FACE_OUTER_BOUND('',#1243,.T.);
#856=FACE_OUTER_BOUND('',#1244,.T.);
#857=FACE_OUTER_BOUND('',#1245,.T.);
#858=FACE_OUTER_BOUND('',#1246,.T.);
#859=FACE_OUTER_BOUND('',#1248,.T.);
#860=FACE_OUTER_BOUND('',#1249,.T.);
#861=FACE_OUTER_BOUND('',#1250,.T.);
#862=FACE_OUTER_BOUND('',#1251,.T.);
#863=FACE_OUTER_BOUND('',#1252,.T.);
#864=FACE_OUTER_BOUND('',#1253,.T.);
#865=FACE_OUTER_BOUND('',#1254,.T.);
#866=FACE_OUTER_BOUND('',#1255,.T.);
#867=FACE_OUTER_BOUND('',#1259,.T.);
#868=FACE_OUTER_BOUND('',#1260,.T.);
#869=FACE_OUTER_BOUND('',#1261,.T.);
#870=FACE_OUTER_BOUND('',#1262,.T.);
#871=FACE_OUTER_BOUND('',#1263,.T.);
#872=FACE_OUTER_BOUND('',#1264,.T.);
#873=FACE_OUTER_BOUND('',#1265,.T.);
#874=FACE_OUTER_BOUND('',#1266,.T.);
#875=FACE_OUTER_BOUND('',#1267,.T.);
#876=FACE_OUTER_BOUND('',#1268,.T.);
#877=FACE_OUTER_BOUND('',#1269,.T.);
#878=FACE_OUTER_BOUND('',#1270,.T.);
#879=FACE_OUTER_BOUND('',#1271,.T.);
#880=FACE_OUTER_BOUND('',#1272,.T.);
#881=FACE_OUTER_BOUND('',#1276,.T.);
#882=FACE_OUTER_BOUND('',#1277,.T.);
#883=FACE_OUTER_BOUND('',#1278,.T.);
#884=FACE_OUTER_BOUND('',#1279,.T.);
#885=FACE_OUTER_BOUND('',#1280,.T.);
#886=FACE_OUTER_BOUND('',#1281,.T.);
#887=FACE_OUTER_BOUND('',#1282,.T.);
#888=FACE_OUTER_BOUND('',#1283,.T.);
#889=FACE_OUTER_BOUND('',#1284,.T.);
#890=FACE_OUTER_BOUND('',#1285,.T.);
#891=FACE_OUTER_BOUND('',#1286,.T.);
#892=FACE_OUTER_BOUND('',#1287,.T.);
#893=FACE_OUTER_BOUND('',#1288,.T.);
#894=FACE_OUTER_BOUND('',#1289,.T.);
#895=FACE_OUTER_BOUND('',#1290,.T.);
#896=FACE_OUTER_BOUND('',#1291,.T.);
#897=FACE_OUTER_BOUND('',#1292,.T.);
#898=FACE_OUTER_BOUND('',#1293,.T.);
#899=FACE_OUTER_BOUND('',#1294,.T.);
#900=FACE_OUTER_BOUND('',#1295,.T.);
#901=FACE_OUTER_BOUND('',#1296,.T.);
#902=FACE_OUTER_BOUND('',#1297,.T.);
#903=FACE_OUTER_BOUND('',#1298,.T.);
#904=FACE_OUTER_BOUND('',#1299,.T.);
#905=FACE_OUTER_BOUND('',#1300,.T.);
#906=FACE_OUTER_BOUND('',#1301,.T.);
#907=FACE_OUTER_BOUND('',#1302,.T.);
#908=FACE_OUTER_BOUND('',#1303,.T.);
#909=FACE_OUTER_BOUND('',#1304,.T.);
#910=FACE_OUTER_BOUND('',#1305,.T.);
#911=FACE_OUTER_BOUND('',#1306,.T.);
#912=FACE_OUTER_BOUND('',#1307,.T.);
#913=FACE_OUTER_BOUND('',#1308,.T.);
#914=FACE_OUTER_BOUND('',#1309,.T.);
#915=FACE_OUTER_BOUND('',#1310,.T.);
#916=FACE_OUTER_BOUND('',#1317,.T.);
#917=FACE_OUTER_BOUND('',#1318,.T.);
#1213=EDGE_LOOP('',(#4330,#4331,#4332,#4333));
#1214=EDGE_LOOP('',(#4334,#4335,#4336,#4337));
#1215=EDGE_LOOP('',(#4338,#4339,#4340,#4341));
#1216=EDGE_LOOP('',(#4342,#4343,#4344,#4345));
#1217=EDGE_LOOP('',(#4346,#4347,#4348,#4349));
#1218=EDGE_LOOP('',(#4350));
#1219=EDGE_LOOP('',(#4351));
#1220=EDGE_LOOP('',(#4352,#4353,#4354,#4355));
#1221=EDGE_LOOP('',(#4356));
#1222=EDGE_LOOP('',(#4357));
#1223=EDGE_LOOP('',(#4358,#4359,#4360,#4361));
#1224=EDGE_LOOP('',(#4362,#4363,#4364,#4365));
#1225=EDGE_LOOP('',(#4366,#4367,#4368,#4369));
#1226=EDGE_LOOP('',(#4370,#4371,#4372,#4373));
#1227=EDGE_LOOP('',(#4374,#4375,#4376,#4377));
#1228=EDGE_LOOP('',(#4378,#4379,#4380,#4381));
#1229=EDGE_LOOP('',(#4382,#4383,#4384,#4385));
#1230=EDGE_LOOP('',(#4386,#4387,#4388,#4389));
#1231=EDGE_LOOP('',(#4390,#4391,#4392,#4393));
#1232=EDGE_LOOP('',(#4394));
#1233=EDGE_LOOP('',(#4395));
#1234=EDGE_LOOP('',(#4396));
#1235=EDGE_LOOP('',(#4397));
#1236=EDGE_LOOP('',(#4398,#4399,#4400,#4401));
#1237=EDGE_LOOP('',(#4402,#4403,#4404,#4405));
#1238=EDGE_LOOP('',(#4406,#4407,#4408,#4409));
#1239=EDGE_LOOP('',(#4410,#4411,#4412,#4413));
#1240=EDGE_LOOP('',(#4414,#4415,#4416,#4417));
#1241=EDGE_LOOP('',(#4418,#4419,#4420,#4421,#4422,#4423));
#1242=EDGE_LOOP('',(#4424,#4425,#4426,#4427,#4428,#4429,#4430,#4431,#4432,
#4433));
#1243=EDGE_LOOP('',(#4434,#4435,#4436,#4437,#4438,#4439,#4440,#4441,#4442,
#4443));
#1244=EDGE_LOOP('',(#4444,#4445,#4446,#4447,#4448,#4449,#4450,#4451,#4452,
#4453));
#1245=EDGE_LOOP('',(#4454,#4455,#4456,#4457,#4458,#4459,#4460,#4461));
#1246=EDGE_LOOP('',(#4462,#4463,#4464,#4465,#4466,#4467,#4468,#4469,#4470,
#4471,#4472,#4473,#4474,#4475,#4476,#4477,#4478,#4479,#4480,#4481,#4482,
#4483,#4484,#4485,#4486,#4487,#4488,#4489,#4490,#4491,#4492,#4493,#4494,
#4495,#4496,#4497,#4498,#4499,#4500,#4501,#4502,#4503));
#1247=EDGE_LOOP('',(#4504,#4505,#4506,#4507,#4508,#4509));
#1248=EDGE_LOOP('',(#4510,#4511,#4512,#4513));
#1249=EDGE_LOOP('',(#4514,#4515,#4516,#4517));
#1250=EDGE_LOOP('',(#4518,#4519,#4520,#4521,#4522,#4523));
#1251=EDGE_LOOP('',(#4524,#4525,#4526,#4527));
#1252=EDGE_LOOP('',(#4528,#4529,#4530,#4531));
#1253=EDGE_LOOP('',(#4532,#4533,#4534,#4535));
#1254=EDGE_LOOP('',(#4536,#4537,#4538,#4539));
#1255=EDGE_LOOP('',(#4540,#4541,#4542,#4543));
#1256=EDGE_LOOP('',(#4544));
#1257=EDGE_LOOP('',(#4545));
#1258=EDGE_LOOP('',(#4546));
#1259=EDGE_LOOP('',(#4547,#4548,#4549,#4550));
#1260=EDGE_LOOP('',(#4551,#4552,#4553,#4554));
#1261=EDGE_LOOP('',(#4555,#4556,#4557,#4558));
#1262=EDGE_LOOP('',(#4559,#4560,#4561,#4562));
#1263=EDGE_LOOP('',(#4563,#4564,#4565,#4566,#4567,#4568,#4569,#4570,#4571,
#4572));
#1264=EDGE_LOOP('',(#4573,#4574,#4575,#4576));
#1265=EDGE_LOOP('',(#4577,#4578,#4579,#4580));
#1266=EDGE_LOOP('',(#4581,#4582,#4583,#4584));
#1267=EDGE_LOOP('',(#4585,#4586,#4587,#4588));
#1268=EDGE_LOOP('',(#4589,#4590,#4591,#4592));
#1269=EDGE_LOOP('',(#4593,#4594,#4595,#4596,#4597,#4598,#4599,#4600,#4601,
#4602));
#1270=EDGE_LOOP('',(#4603,#4604,#4605,#4606));
#1271=EDGE_LOOP('',(#4607,#4608,#4609,#4610));
#1272=EDGE_LOOP('',(#4611,#4612,#4613,#4614));
#1273=EDGE_LOOP('',(#4615));
#1274=EDGE_LOOP('',(#4616));
#1275=EDGE_LOOP('',(#4617));
#1276=EDGE_LOOP('',(#4618,#4619,#4620,#4621));
#1277=EDGE_LOOP('',(#4622,#4623,#4624,#4625));
#1278=EDGE_LOOP('',(#4626,#4627,#4628,#4629,#4630,#4631,#4632,#4633,#4634,
#4635));
#1279=EDGE_LOOP('',(#4636,#4637,#4638,#4639));
#1280=EDGE_LOOP('',(#4640,#4641,#4642,#4643));
#1281=EDGE_LOOP('',(#4644,#4645,#4646,#4647));
#1282=EDGE_LOOP('',(#4648,#4649,#4650,#4651));
#1283=EDGE_LOOP('',(#4652,#4653,#4654,#4655));
#1284=EDGE_LOOP('',(#4656,#4657,#4658));
#1285=EDGE_LOOP('',(#4659,#4660,#4661));
#1286=EDGE_LOOP('',(#4662,#4663,#4664));
#1287=EDGE_LOOP('',(#4665,#4666,#4667,#4668));
#1288=EDGE_LOOP('',(#4669,#4670,#4671,#4672));
#1289=EDGE_LOOP('',(#4673,#4674,#4675));
#1290=EDGE_LOOP('',(#4676,#4677,#4678,#4679));
#1291=EDGE_LOOP('',(#4680,#4681,#4682,#4683));
#1292=EDGE_LOOP('',(#4684,#4685,#4686,#4687));
#1293=EDGE_LOOP('',(#4688,#4689,#4690,#4691));
#1294=EDGE_LOOP('',(#4692,#4693,#4694,#4695));
#1295=EDGE_LOOP('',(#4696,#4697,#4698,#4699));
#1296=EDGE_LOOP('',(#4700,#4701,#4702));
#1297=EDGE_LOOP('',(#4703,#4704,#4705));
#1298=EDGE_LOOP('',(#4706,#4707,#4708));
#1299=EDGE_LOOP('',(#4709,#4710,#4711,#4712));
#1300=EDGE_LOOP('',(#4713,#4714,#4715,#4716));
#1301=EDGE_LOOP('',(#4717,#4718,#4719));
#1302=EDGE_LOOP('',(#4720,#4721,#4722,#4723));
#1303=EDGE_LOOP('',(#4724,#4725,#4726,#4727));
#1304=EDGE_LOOP('',(#4728,#4729,#4730,#4731));
#1305=EDGE_LOOP('',(#4732,#4733,#4734,#4735));
#1306=EDGE_LOOP('',(#4736,#4737,#4738,#4739));
#1307=EDGE_LOOP('',(#4740,#4741,#4742,#4743));
#1308=EDGE_LOOP('',(#4744,#4745,#4746,#4747));
#1309=EDGE_LOOP('',(#4748,#4749,#4750,#4751,#4752,#4753,#4754,#4755));
#1310=EDGE_LOOP('',(#4756,#4757,#4758,#4759));
#1311=EDGE_LOOP('',(#4760));
#1312=EDGE_LOOP('',(#4761));
#1313=EDGE_LOOP('',(#4762));
#1314=EDGE_LOOP('',(#4763));
#1315=EDGE_LOOP('',(#4764));
#1316=EDGE_LOOP('',(#4765));
#1317=EDGE_LOOP('',(#4766,#4767,#4768,#4769));
#1318=EDGE_LOOP('',(#4770,#4771,#4772,#4773));
#1663=LINE('',#8701,#2067);
#1664=LINE('',#8707,#2068);
#1665=LINE('',#8713,#2069);
#1666=LINE('',#8719,#2070);
#1667=LINE('',#8725,#2071);
#1668=LINE('',#8734,#2072);
#1669=LINE('',#8741,#2073);
#1670=LINE('',#8745,#2074);
#1671=LINE('',#8750,#2075);
#1672=LINE('',#8752,#2076);
#1673=LINE('',#8754,#2077);
#1674=LINE('',#8755,#2078);
#1675=LINE('',#8759,#2079);
#1676=LINE('',#8761,#2080);
#1677=LINE('',#8763,#2081);
#1678=LINE('',#8764,#2082);
#1679=LINE('',#8768,#2083);
#1680=LINE('',#8770,#2084);
#1681=LINE('',#8772,#2085);
#1682=LINE('',#8773,#2086);
#1683=LINE('',#8777,#2087);
#1684=LINE('',#8779,#2088);
#1685=LINE('',#8781,#2089);
#1686=LINE('',#8782,#2090);
#1687=LINE('',#8786,#2091);
#1688=LINE('',#8788,#2092);
#1689=LINE('',#8790,#2093);
#1690=LINE('',#8791,#2094);
#1691=LINE('',#8795,#2095);
#1692=LINE('',#8797,#2096);
#1693=LINE('',#8799,#2097);
#1694=LINE('',#8800,#2098);
#1695=LINE('',#8804,#2099);
#1696=LINE('',#8806,#2100);
#1697=LINE('',#8808,#2101);
#1698=LINE('',#8809,#2102);
#1699=LINE('',#8817,#2103);
#1700=LINE('',#8818,#2104);
#1701=LINE('',#8820,#2105);
#1702=LINE('',#8821,#2106);
#1703=LINE('',#8823,#2107);
#1704=LINE('',#8824,#2108);
#1705=LINE('',#8827,#2109);
#1706=LINE('',#8829,#2110);
#1707=LINE('',#8830,#2111);
#1708=LINE('',#8833,#2112);
#1709=LINE('',#8835,#2113);
#1710=LINE('',#8836,#2114);
#1711=LINE('',#8840,#2115);
#1712=LINE('',#8878,#2116);
#1713=LINE('',#8916,#2117);
#1714=LINE('',#8954,#2118);
#1715=LINE('',#8991,#2119);
#1716=LINE('',#8994,#2120);
#1717=LINE('',#9032,#2121);
#1718=LINE('',#9069,#2122);
#1719=LINE('',#9072,#2123);
#1720=LINE('',#9110,#2124);
#1721=LINE('',#9147,#2125);
#1722=LINE('',#9150,#2126);
#1723=LINE('',#9157,#2127);
#1724=LINE('',#9163,#2128);
#1725=LINE('',#9180,#2129);
#1726=LINE('',#9189,#2130);
#1727=LINE('',#9195,#2131);
#1728=LINE('',#9230,#2132);
#1729=LINE('',#9301,#2133);
#1730=LINE('',#9371,#2134);
#1731=LINE('',#9406,#2135);
#1732=LINE('',#9412,#2136);
#1733=LINE('',#9421,#2137);
#1734=LINE('',#9455,#2138);
#1735=LINE('',#9487,#2139);
#1736=LINE('',#9491,#2140);
#1737=LINE('',#9495,#2141);
#1738=LINE('',#9541,#2142);
#1739=LINE('',#9676,#2143);
#1740=LINE('',#9780,#2144);
#1741=LINE('',#9943,#2145);
#1742=LINE('',#10106,#2146);
#1743=LINE('',#10195,#2147);
#1744=LINE('',#10283,#2148);
#1745=LINE('',#10395,#2149);
#1746=LINE('',#10396,#2150);
#1747=LINE('',#10433,#2151);
#1748=LINE('',#10434,#2152);
#2067=VECTOR('',#7342,0.15);
#2068=VECTOR('',#7349,0.15);
#2069=VECTOR('',#7356,0.15);
#2070=VECTOR('',#7363,0.15);
#2071=VECTOR('',#7370,0.3);
#2072=VECTOR('',#7381,0.3);
#2073=VECTOR('',#7390,0.17);
#2074=VECTOR('',#7395,0.17);
#2075=VECTOR('',#7400,1.);
#2076=VECTOR('',#7401,1.);
#2077=VECTOR('',#7402,1.);
#2078=VECTOR('',#7403,1.);
#2079=VECTOR('',#7406,1.);
#2080=VECTOR('',#7407,1.);
#2081=VECTOR('',#7408,1.);
#2082=VECTOR('',#7409,1.);
#2083=VECTOR('',#7412,1.);
#2084=VECTOR('',#7413,1.);
#2085=VECTOR('',#7414,1.);
#2086=VECTOR('',#7415,1.);
#2087=VECTOR('',#7418,1.);
#2088=VECTOR('',#7419,1.);
#2089=VECTOR('',#7420,1.);
#2090=VECTOR('',#7421,1.);
#2091=VECTOR('',#7424,1.);
#2092=VECTOR('',#7425,1.);
#2093=VECTOR('',#7426,1.);
#2094=VECTOR('',#7427,1.);
#2095=VECTOR('',#7430,1.);
#2096=VECTOR('',#7431,1.);
#2097=VECTOR('',#7432,1.);
#2098=VECTOR('',#7433,1.);
#2099=VECTOR('',#7436,1.);
#2100=VECTOR('',#7437,1.);
#2101=VECTOR('',#7438,1.);
#2102=VECTOR('',#7439,1.);
#2103=VECTOR('',#7450,1.);
#2104=VECTOR('',#7451,1.);
#2105=VECTOR('',#7454,1.);
#2106=VECTOR('',#7455,1.);
#2107=VECTOR('',#7458,1.);
#2108=VECTOR('',#7459,1.);
#2109=VECTOR('',#7462,1.);
#2110=VECTOR('',#7463,1.);
#2111=VECTOR('',#7464,1.);
#2112=VECTOR('',#7467,1.);
#2113=VECTOR('',#7468,1.);
#2114=VECTOR('',#7469,1.);
#2115=VECTOR('',#7472,1.);
#2116=VECTOR('',#7473,1.);
#2117=VECTOR('',#7476,1.);
#2118=VECTOR('',#7477,1.);
#2119=VECTOR('',#7478,1.);
#2120=VECTOR('',#7481,1.);
#2121=VECTOR('',#7482,1.);
#2122=VECTOR('',#7483,1.);
#2123=VECTOR('',#7486,1.);
#2124=VECTOR('',#7487,1.);
#2125=VECTOR('',#7488,1.);
#2126=VECTOR('',#7491,1.);
#2127=VECTOR('',#7492,1.);
#2128=VECTOR('',#7493,1.);
#2129=VECTOR('',#7496,1.);
#2130=VECTOR('',#7497,1.);
#2131=VECTOR('',#7498,1.);
#2132=VECTOR('',#7499,1.);
#2133=VECTOR('',#7500,1.);
#2134=VECTOR('',#7501,1.);
#2135=VECTOR('',#7502,1.);
#2136=VECTOR('',#7503,1.);
#2137=VECTOR('',#7504,1.);
#2138=VECTOR('',#7505,1.);
#2139=VECTOR('',#7506,1.);
#2140=VECTOR('',#7511,0.4);
#2141=VECTOR('',#7516,0.4);
#2142=VECTOR('',#7519,1.);
#2143=VECTOR('',#7526,1.);
#2144=VECTOR('',#7529,1.);
#2145=VECTOR('',#7534,1.);
#2146=VECTOR('',#7539,1.);
#2147=VECTOR('',#7544,1.);
#2148=VECTOR('',#7577,1.);
#2149=VECTOR('',#7606,1.);
#2150=VECTOR('',#7607,1.);
#2151=VECTOR('',#7618,1.);
#2152=VECTOR('',#7619,1.);
#2438=CIRCLE('',#6688,0.15);
#2439=CIRCLE('',#6689,0.15);
#2440=CIRCLE('',#6691,0.15);
#2441=CIRCLE('',#6692,0.15);
#2442=CIRCLE('',#6694,0.15);
#2443=CIRCLE('',#6695,0.15);
#2444=CIRCLE('',#6697,0.15);
#2445=CIRCLE('',#6698,0.15);
#2446=CIRCLE('',#6700,0.3);
#2447=CIRCLE('',#6701,0.3);
#2448=CIRCLE('',#6703,0.17);
#2449=CIRCLE('',#6705,0.3);
#2450=CIRCLE('',#6706,0.3);
#2451=CIRCLE('',#6708,0.17);
#2452=CIRCLE('',#6710,0.17);
#2453=CIRCLE('',#6712,0.17);
#2454=CIRCLE('',#6721,0.4);
#2455=CIRCLE('',#6723,0.4);
#2456=CIRCLE('',#6736,0.4);
#2457=CIRCLE('',#6738,0.4);
#2458=CIRCLE('',#6740,0.1);
#2459=CIRCLE('',#6748,0.0999999999999994);
#2460=CIRCLE('',#6750,0.0999999999999999);
#2461=CIRCLE('',#6752,0.1);
#2462=CIRCLE('',#6753,0.1);
#2463=CIRCLE('',#6755,0.100000000000001);
#2464=CIRCLE('',#6756,0.100000000000001);
#2465=CIRCLE('',#6757,0.100000000000002);
#2466=CIRCLE('',#6759,0.0999999999999995);
#2467=CIRCLE('',#6760,0.0999999999999991);
#2468=CIRCLE('',#6763,0.100000000000001);
#2469=CIRCLE('',#6764,0.1);
#2470=CIRCLE('',#6768,0.3);
#2471=CIRCLE('',#6769,0.3);
#2472=CIRCLE('',#6770,0.3);
#2473=CIRCLE('',#6772,0.3);
#2474=CIRCLE('',#6773,0.300000000000002);
#2475=CIRCLE('',#6774,0.3);
#2476=CIRCLE('',#6776,0.3);
#2477=CIRCLE('',#6777,0.299999999999999);
#2478=CIRCLE('',#6778,0.3);
#2479=CIRCLE('',#6781,0.300000000000001);
#2480=CIRCLE('',#6782,0.3);
#2481=CIRCLE('',#6783,0.3);
#2639=VERTEX_POINT('',#8698);
#2640=VERTEX_POINT('',#8700);
#2641=VERTEX_POINT('',#8704);
#2642=VERTEX_POINT('',#8706);
#2643=VERTEX_POINT('',#8710);
#2644=VERTEX_POINT('',#8712);
#2645=VERTEX_POINT('',#8716);
#2646=VERTEX_POINT('',#8718);
#2647=VERTEX_POINT('',#8722);
#2648=VERTEX_POINT('',#8724);
#2649=VERTEX_POINT('',#8728);
#2650=VERTEX_POINT('',#8731);
#2651=VERTEX_POINT('',#8733);
#2652=VERTEX_POINT('',#8737);
#2653=VERTEX_POINT('',#8740);
#2654=VERTEX_POINT('',#8744);
#2655=VERTEX_POINT('',#8748);
#2656=VERTEX_POINT('',#8749);
#2657=VERTEX_POINT('',#8751);
#2658=VERTEX_POINT('',#8753);
#2659=VERTEX_POINT('',#8757);
#2660=VERTEX_POINT('',#8758);
#2661=VERTEX_POINT('',#8760);
#2662=VERTEX_POINT('',#8762);
#2663=VERTEX_POINT('',#8766);
#2664=VERTEX_POINT('',#8767);
#2665=VERTEX_POINT('',#8769);
#2666=VERTEX_POINT('',#8771);
#2667=VERTEX_POINT('',#8775);
#2668=VERTEX_POINT('',#8776);
#2669=VERTEX_POINT('',#8778);
#2670=VERTEX_POINT('',#8780);
#2671=VERTEX_POINT('',#8784);
#2672=VERTEX_POINT('',#8785);
#2673=VERTEX_POINT('',#8787);
#2674=VERTEX_POINT('',#8789);
#2675=VERTEX_POINT('',#8793);
#2676=VERTEX_POINT('',#8794);
#2677=VERTEX_POINT('',#8796);
#2678=VERTEX_POINT('',#8798);
#2679=VERTEX_POINT('',#8802);
#2680=VERTEX_POINT('',#8803);
#2681=VERTEX_POINT('',#8805);
#2682=VERTEX_POINT('',#8807);
#2683=VERTEX_POINT('',#8811);
#2684=VERTEX_POINT('',#8814);
#2685=VERTEX_POINT('',#8826);
#2686=VERTEX_POINT('',#8828);
#2687=VERTEX_POINT('',#8832);
#2688=VERTEX_POINT('',#8834);
#2689=VERTEX_POINT('',#8838);
#2690=VERTEX_POINT('',#8839);
#2691=VERTEX_POINT('',#8841);
#2692=VERTEX_POINT('',#8848);
#2693=VERTEX_POINT('',#8877);
#2694=VERTEX_POINT('',#8879);
#2695=VERTEX_POINT('',#8915);
#2696=VERTEX_POINT('',#8917);
#2697=VERTEX_POINT('',#8924);
#2698=VERTEX_POINT('',#8953);
#2699=VERTEX_POINT('',#8955);
#2700=VERTEX_POINT('',#8984);
#2701=VERTEX_POINT('',#8993);
#2702=VERTEX_POINT('',#8995);
#2703=VERTEX_POINT('',#9002);
#2704=VERTEX_POINT('',#9031);
#2705=VERTEX_POINT('',#9033);
#2706=VERTEX_POINT('',#9062);
#2707=VERTEX_POINT('',#9071);
#2708=VERTEX_POINT('',#9073);
#2709=VERTEX_POINT('',#9080);
#2710=VERTEX_POINT('',#9109);
#2711=VERTEX_POINT('',#9111);
#2712=VERTEX_POINT('',#9140);
#2713=VERTEX_POINT('',#9149);
#2714=VERTEX_POINT('',#9151);
#2715=VERTEX_POINT('',#9156);
#2716=VERTEX_POINT('',#9158);
#2717=VERTEX_POINT('',#9179);
#2718=VERTEX_POINT('',#9188);
#2719=VERTEX_POINT('',#9194);
#2720=VERTEX_POINT('',#9196);
#2721=VERTEX_POINT('',#9229);
#2722=VERTEX_POINT('',#9231);
#2723=VERTEX_POINT('',#9263);
#2724=VERTEX_POINT('',#9268);
#2725=VERTEX_POINT('',#9300);
#2726=VERTEX_POINT('',#9302);
#2727=VERTEX_POINT('',#9334);
#2728=VERTEX_POINT('',#9339);
#2729=VERTEX_POINT('',#9372);
#2730=VERTEX_POINT('',#9401);
#2731=VERTEX_POINT('',#9407);
#2732=VERTEX_POINT('',#9413);
#2733=VERTEX_POINT('',#9422);
#2734=VERTEX_POINT('',#9423);
#2735=VERTEX_POINT('',#9428);
#2736=VERTEX_POINT('',#9454);
#2737=VERTEX_POINT('',#9456);
#2738=VERTEX_POINT('',#9482);
#2739=VERTEX_POINT('',#9489);
#2740=VERTEX_POINT('',#9493);
#2741=VERTEX_POINT('',#9497);
#2742=VERTEX_POINT('',#9504);
#2743=VERTEX_POINT('',#9511);
#2744=VERTEX_POINT('',#9540);
#2745=VERTEX_POINT('',#9606);
#2746=VERTEX_POINT('',#9659);
#2747=VERTEX_POINT('',#9671);
#2748=VERTEX_POINT('',#9733);
#2749=VERTEX_POINT('',#9743);
#2750=VERTEX_POINT('',#9750);
#2751=VERTEX_POINT('',#9779);
#2752=VERTEX_POINT('',#9781);
#2753=VERTEX_POINT('',#9906);
#2754=VERTEX_POINT('',#9913);
#2755=VERTEX_POINT('',#9942);
#2756=VERTEX_POINT('',#9944);
#2757=VERTEX_POINT('',#10069);
#2758=VERTEX_POINT('',#10076);
#2759=VERTEX_POINT('',#10105);
#2760=VERTEX_POINT('',#10107);
#2761=VERTEX_POINT('',#10158);
#2762=VERTEX_POINT('',#10187);
#2763=VERTEX_POINT('',#10194);
#2764=VERTEX_POINT('',#10216);
#2765=VERTEX_POINT('',#10251);
#2766=VERTEX_POINT('',#10279);
#2767=VERTEX_POINT('',#10374);
#2768=VERTEX_POINT('',#10375);
#2769=VERTEX_POINT('',#10377);
#2770=VERTEX_POINT('',#10381);
#2771=VERTEX_POINT('',#10382);
#2772=VERTEX_POINT('',#10384);
#2773=VERTEX_POINT('',#10388);
#2774=VERTEX_POINT('',#10389);
#2775=VERTEX_POINT('',#10391);
#2776=VERTEX_POINT('',#10426);
#2777=VERTEX_POINT('',#10427);
#2778=VERTEX_POINT('',#10429);
#3282=EDGE_CURVE('',#2639,#2639,#2438,.T.);
#3283=EDGE_CURVE('',#2639,#2640,#1663,.T.);
#3284=EDGE_CURVE('',#2640,#2640,#2439,.T.);
#3285=EDGE_CURVE('',#2641,#2641,#2440,.T.);
#3286=EDGE_CURVE('',#2641,#2642,#1664,.T.);
#3287=EDGE_CURVE('',#2642,#2642,#2441,.T.);
#3288=EDGE_CURVE('',#2643,#2643,#2442,.T.);
#3289=EDGE_CURVE('',#2643,#2644,#1665,.T.);
#3290=EDGE_CURVE('',#2644,#2644,#2443,.T.);
#3291=EDGE_CURVE('',#2645,#2645,#2444,.T.);
#3292=EDGE_CURVE('',#2645,#2646,#1666,.T.);
#3293=EDGE_CURVE('',#2646,#2646,#2445,.T.);
#3294=EDGE_CURVE('',#2647,#2647,#2446,.T.);
#3295=EDGE_CURVE('',#2647,#2648,#1667,.T.);
#3296=EDGE_CURVE('',#2648,#2648,#2447,.T.);
#3297=EDGE_CURVE('',#2649,#2649,#2448,.T.);
#3298=EDGE_CURVE('',#2650,#2650,#2449,.T.);
#3299=EDGE_CURVE('',#2650,#2651,#1668,.T.);
#3300=EDGE_CURVE('',#2651,#2651,#2450,.T.);
#3301=EDGE_CURVE('',#2652,#2652,#2451,.T.);
#3302=EDGE_CURVE('',#2649,#2653,#1669,.T.);
#3303=EDGE_CURVE('',#2653,#2653,#2452,.T.);
#3304=EDGE_CURVE('',#2652,#2654,#1670,.T.);
#3305=EDGE_CURVE('',#2654,#2654,#2453,.T.);
#3306=EDGE_CURVE('',#2655,#2656,#1671,.T.);
#3307=EDGE_CURVE('',#2657,#2655,#1672,.T.);
#3308=EDGE_CURVE('',#2658,#2657,#1673,.T.);
#3309=EDGE_CURVE('',#2658,#2656,#1674,.T.);
#3310=EDGE_CURVE('',#2659,#2660,#1675,.T.);
#3311=EDGE_CURVE('',#2659,#2661,#1676,.T.);
#3312=EDGE_CURVE('',#2662,#2661,#1677,.T.);
#3313=EDGE_CURVE('',#2660,#2662,#1678,.T.);
#3314=EDGE_CURVE('',#2663,#2664,#1679,.T.);
#3315=EDGE_CURVE('',#2663,#2665,#1680,.T.);
#3316=EDGE_CURVE('',#2666,#2665,#1681,.T.);
#3317=EDGE_CURVE('',#2664,#2666,#1682,.T.);
#3318=EDGE_CURVE('',#2667,#2668,#1683,.T.);
#3319=EDGE_CURVE('',#2667,#2669,#1684,.T.);
#3320=EDGE_CURVE('',#2670,#2669,#1685,.T.);
#3321=EDGE_CURVE('',#2668,#2670,#1686,.T.);
#3322=EDGE_CURVE('',#2671,#2672,#1687,.T.);
#3323=EDGE_CURVE('',#2671,#2673,#1688,.T.);
#3324=EDGE_CURVE('',#2674,#2673,#1689,.T.);
#3325=EDGE_CURVE('',#2672,#2674,#1690,.T.);
#3326=EDGE_CURVE('',#2675,#2676,#1691,.T.);
#3327=EDGE_CURVE('',#2677,#2675,#1692,.T.);
#3328=EDGE_CURVE('',#2678,#2677,#1693,.T.);
#3329=EDGE_CURVE('',#2678,#2676,#1694,.T.);
#3330=EDGE_CURVE('',#2679,#2680,#1695,.T.);
#3331=EDGE_CURVE('',#2681,#2679,#1696,.T.);
#3332=EDGE_CURVE('',#2682,#2681,#1697,.T.);
#3333=EDGE_CURVE('',#2682,#2680,#1698,.T.);
#3334=EDGE_CURVE('',#2683,#2683,#2454,.T.);
#3335=EDGE_CURVE('',#2684,#2684,#2455,.T.);
#3336=EDGE_CURVE('',#2656,#2671,#1699,.T.);
#3337=EDGE_CURVE('',#2673,#2658,#1700,.T.);
#3338=EDGE_CURVE('',#2676,#2659,#1701,.T.);
#3339=EDGE_CURVE('',#2661,#2678,#1702,.T.);
#3340=EDGE_CURVE('',#2680,#2663,#1703,.T.);
#3341=EDGE_CURVE('',#2665,#2682,#1704,.T.);
#3342=EDGE_CURVE('',#2685,#2667,#1705,.T.);
#3343=EDGE_CURVE('',#2686,#2685,#1706,.T.);
#3344=EDGE_CURVE('',#2669,#2686,#1707,.T.);
#3345=EDGE_CURVE('',#2687,#2685,#1708,.T.);
#3346=EDGE_CURVE('',#2688,#2687,#1709,.T.);
#3347=EDGE_CURVE('',#2686,#2688,#1710,.T.);
#3348=EDGE_CURVE('',#2689,#2690,#1711,.T.);
#3349=EDGE_CURVE('',#2691,#2690,#171,.T.);
#3350=EDGE_CURVE('',#2692,#2691,#172,.T.);
#3351=EDGE_CURVE('',#2693,#2692,#1712,.T.);
#3352=EDGE_CURVE('',#2694,#2693,#173,.T.);
#3353=EDGE_CURVE('',#2689,#2694,#174,.T.);
#3354=EDGE_CURVE('',#2688,#2695,#1713,.T.);
#3355=EDGE_CURVE('',#2696,#2695,#175,.T.);
#3356=EDGE_CURVE('',#2697,#2696,#176,.T.);
#3357=EDGE_CURVE('',#2698,#2697,#1714,.T.);
#3358=EDGE_CURVE('',#2699,#2698,#177,.T.);
#3359=EDGE_CURVE('',#2700,#2699,#178,.T.);
#3360=EDGE_CURVE('',#2700,#2670,#1715,.T.);
#3361=EDGE_CURVE('',#2681,#2701,#1716,.T.);
#3362=EDGE_CURVE('',#2702,#2701,#179,.T.);
#3363=EDGE_CURVE('',#2703,#2702,#180,.T.);
#3364=EDGE_CURVE('',#2704,#2703,#1717,.T.);
#3365=EDGE_CURVE('',#2705,#2704,#181,.T.);
#3366=EDGE_CURVE('',#2706,#2705,#182,.T.);
#3367=EDGE_CURVE('',#2706,#2666,#1718,.T.);
#3368=EDGE_CURVE('',#2677,#2707,#1719,.T.);
#3369=EDGE_CURVE('',#2708,#2707,#183,.T.);
#3370=EDGE_CURVE('',#2709,#2708,#184,.T.);
#3371=EDGE_CURVE('',#2710,#2709,#1720,.T.);
#3372=EDGE_CURVE('',#2711,#2710,#185,.T.);
#3373=EDGE_CURVE('',#2712,#2711,#186,.T.);
#3374=EDGE_CURVE('',#2712,#2662,#1721,.T.);
#3375=EDGE_CURVE('',#2713,#2672,#1722,.T.);
#3376=EDGE_CURVE('',#2713,#2714,#187,.T.);
#3377=EDGE_CURVE('',#2714,#2715,#1723,.T.);
#3378=EDGE_CURVE('',#2715,#2716,#188,.T.);
#3379=EDGE_CURVE('',#2655,#2716,#1724,.T.);
#3380=EDGE_CURVE('',#2700,#2690,#189,.T.);
#3381=EDGE_CURVE('',#2689,#2695,#190,.T.);
#3382=EDGE_CURVE('',#2717,#2687,#1725,.T.);
#3383=EDGE_CURVE('',#2717,#2701,#191,.T.);
#3384=EDGE_CURVE('',#2718,#2679,#1726,.T.);
#3385=EDGE_CURVE('',#2718,#2707,#192,.T.);
#3386=EDGE_CURVE('',#2719,#2675,#1727,.T.);
#3387=EDGE_CURVE('',#2719,#2720,#193,.T.);
#3388=EDGE_CURVE('',#2720,#2713,#194,.T.);
#3389=EDGE_CURVE('',#2674,#2721,#1728,.T.);
#3390=EDGE_CURVE('',#2722,#2721,#195,.T.);
#3391=EDGE_CURVE('',#2722,#2723,#196,.T.);
#3392=EDGE_CURVE('',#2724,#2723,#197,.T.);
#3393=EDGE_CURVE('',#2724,#2725,#1729,.T.);
#3394=EDGE_CURVE('',#2726,#2725,#198,.T.);
#3395=EDGE_CURVE('',#2726,#2727,#199,.T.);
#3396=EDGE_CURVE('',#2728,#2727,#200,.T.);
#3397=EDGE_CURVE('',#2728,#2657,#1730,.T.);
#3398=EDGE_CURVE('',#2716,#2729,#201,.T.);
#3399=EDGE_CURVE('',#2729,#2730,#202,.T.);
#3400=EDGE_CURVE('',#2660,#2730,#1731,.T.);
#3401=EDGE_CURVE('',#2712,#2731,#203,.T.);
#3402=EDGE_CURVE('',#2664,#2731,#1732,.T.);
#3403=EDGE_CURVE('',#2706,#2732,#204,.T.);
#3404=EDGE_CURVE('',#2668,#2732,#1733,.T.);
#3405=EDGE_CURVE('',#2733,#2734,#205,.T.);
#3406=EDGE_CURVE('',#2734,#2735,#206,.T.);
#3407=EDGE_CURVE('',#2735,#2736,#1734,.T.);
#3408=EDGE_CURVE('',#2736,#2737,#207,.T.);
#3409=EDGE_CURVE('',#2737,#2738,#208,.T.);
#3410=EDGE_CURVE('',#2733,#2738,#1735,.T.);
#3411=EDGE_CURVE('',#2739,#2739,#2456,.T.);
#3412=EDGE_CURVE('',#2739,#2684,#1736,.T.);
#3413=EDGE_CURVE('',#2740,#2740,#2457,.T.);
#3414=EDGE_CURVE('',#2740,#2683,#1737,.T.);
#3415=EDGE_CURVE('',#2733,#2741,#209,.T.);
#3416=EDGE_CURVE('',#2742,#2738,#210,.T.);
#3417=EDGE_CURVE('',#2743,#2742,#211,.T.);
#3418=EDGE_CURVE('',#2744,#2743,#1738,.T.);
#3419=EDGE_CURVE('',#2741,#2744,#212,.T.);
#3420=EDGE_CURVE('',#2699,#2691,#213,.T.);
#3421=EDGE_CURVE('',#2741,#2745,#214,.T.);
#3422=EDGE_CURVE('',#2745,#2734,#215,.T.);
#3423=EDGE_CURVE('',#2692,#2698,#216,.T.);
#3424=EDGE_CURVE('',#2746,#2744,#217,.T.);
#3425=EDGE_CURVE('',#2745,#2746,#2458,.F.);
#3426=EDGE_CURVE('',#2697,#2693,#218,.T.);
#3427=EDGE_CURVE('',#2743,#2747,#219,.T.);
#3428=EDGE_CURVE('',#2747,#2746,#1739,.T.);
#3429=EDGE_CURVE('',#2694,#2696,#220,.T.);
#3430=EDGE_CURVE('',#2737,#2748,#221,.T.);
#3431=EDGE_CURVE('',#2748,#2742,#222,.T.);
#3432=EDGE_CURVE('',#2749,#2732,#223,.T.);
#3433=EDGE_CURVE('',#2750,#2749,#224,.T.);
#3434=EDGE_CURVE('',#2751,#2750,#1740,.T.);
#3435=EDGE_CURVE('',#2752,#2751,#225,.T.);
#3436=EDGE_CURVE('',#2717,#2752,#226,.T.);
#3437=EDGE_CURVE('',#2705,#2749,#227,.T.);
#3438=EDGE_CURVE('',#2750,#2704,#228,.T.);
#3439=EDGE_CURVE('',#2703,#2751,#229,.T.);
#3440=EDGE_CURVE('',#2752,#2702,#230,.T.);
#3441=EDGE_CURVE('',#2753,#2731,#231,.T.);
#3442=EDGE_CURVE('',#2754,#2753,#232,.T.);
#3443=EDGE_CURVE('',#2755,#2754,#1741,.T.);
#3444=EDGE_CURVE('',#2756,#2755,#233,.T.);
#3445=EDGE_CURVE('',#2718,#2756,#234,.T.);
#3446=EDGE_CURVE('',#2711,#2753,#235,.T.);
#3447=EDGE_CURVE('',#2754,#2710,#236,.T.);
#3448=EDGE_CURVE('',#2709,#2755,#237,.T.);
#3449=EDGE_CURVE('',#2756,#2708,#238,.T.);
#3450=EDGE_CURVE('',#2757,#2730,#239,.T.);
#3451=EDGE_CURVE('',#2758,#2757,#240,.T.);
#3452=EDGE_CURVE('',#2759,#2758,#1742,.T.);
#3453=EDGE_CURVE('',#2760,#2759,#241,.T.);
#3454=EDGE_CURVE('',#2719,#2760,#242,.T.);
#3455=EDGE_CURVE('',#2729,#2761,#243,.T.);
#3456=EDGE_CURVE('',#2761,#2757,#244,.T.);
#3457=EDGE_CURVE('',#2762,#2761,#2459,.F.);
#3458=EDGE_CURVE('',#2758,#2762,#245,.T.);
#3459=EDGE_CURVE('',#2762,#2763,#1743,.T.);
#3460=EDGE_CURVE('',#2763,#2759,#246,.T.);
#3461=EDGE_CURVE('',#2760,#2764,#247,.T.);
#3462=EDGE_CURVE('',#2764,#2720,#248,.T.);
#3463=EDGE_CURVE('',#2764,#2763,#2460,.F.);
#3464=EDGE_CURVE('',#2763,#2714,#2461,.F.);
#3465=EDGE_CURVE('',#2714,#2764,#2462,.F.);
#3466=EDGE_CURVE('',#2747,#2748,#2463,.F.);
#3467=EDGE_CURVE('',#2748,#2765,#2464,.F.);
#3468=EDGE_CURVE('',#2765,#2747,#2465,.F.);
#3469=EDGE_CURVE('',#2761,#2715,#2466,.F.);
#3470=EDGE_CURVE('',#2715,#2762,#2467,.F.);
#3471=EDGE_CURVE('',#2766,#2745,#2468,.F.);
#3472=EDGE_CURVE('',#2746,#2766,#2469,.F.);
#3473=EDGE_CURVE('',#2766,#2765,#1744,.T.);
#3474=EDGE_CURVE('',#2735,#2766,#249,.T.);
#3475=EDGE_CURVE('',#2765,#2736,#250,.T.);
#3476=EDGE_CURVE('',#2767,#2768,#2470,.F.);
#3477=EDGE_CURVE('',#2769,#2767,#2471,.F.);
#3478=EDGE_CURVE('',#2768,#2769,#2472,.F.);
#3479=EDGE_CURVE('',#2770,#2771,#2473,.F.);
#3480=EDGE_CURVE('',#2772,#2770,#2474,.F.);
#3481=EDGE_CURVE('',#2771,#2772,#2475,.F.);
#3482=EDGE_CURVE('',#2773,#2774,#2476,.F.);
#3483=EDGE_CURVE('',#2775,#2773,#2477,.F.);
#3484=EDGE_CURVE('',#2774,#2775,#2478,.F.);
#3485=EDGE_CURVE('',#2768,#2775,#1745,.T.);
#3486=EDGE_CURVE('',#2773,#2767,#1746,.T.);
#3487=EDGE_CURVE('',#2727,#2774,#251,.T.);
#3488=EDGE_CURVE('',#2775,#2728,#252,.T.);
#3489=EDGE_CURVE('',#2776,#2777,#2479,.F.);
#3490=EDGE_CURVE('',#2778,#2776,#2480,.F.);
#3491=EDGE_CURVE('',#2777,#2778,#2481,.F.);
#3492=EDGE_CURVE('',#2776,#2772,#1747,.T.);
#3493=EDGE_CURVE('',#2770,#2778,#1748,.T.);
#3494=EDGE_CURVE('',#2774,#2777,#253,.T.);
#3495=EDGE_CURVE('',#2778,#2773,#254,.T.);
#3496=EDGE_CURVE('',#2725,#2776,#255,.T.);
#3497=EDGE_CURVE('',#2777,#2726,#256,.T.);
#3498=EDGE_CURVE('',#2723,#2771,#257,.T.);
#3499=EDGE_CURVE('',#2772,#2724,#258,.T.);
#3500=EDGE_CURVE('',#2771,#2769,#259,.T.);
#3501=EDGE_CURVE('',#2767,#2770,#260,.T.);
#3502=EDGE_CURVE('',#2721,#2768,#261,.T.);
#3503=EDGE_CURVE('',#2769,#2722,#262,.T.);
#4330=ORIENTED_EDGE('',*,*,#3282,.F.);
#4331=ORIENTED_EDGE('',*,*,#3283,.T.);
#4332=ORIENTED_EDGE('',*,*,#3284,.F.);
#4333=ORIENTED_EDGE('',*,*,#3283,.F.);
#4334=ORIENTED_EDGE('',*,*,#3285,.F.);
#4335=ORIENTED_EDGE('',*,*,#3286,.T.);
#4336=ORIENTED_EDGE('',*,*,#3287,.F.);
#4337=ORIENTED_EDGE('',*,*,#3286,.F.);
#4338=ORIENTED_EDGE('',*,*,#3288,.F.);
#4339=ORIENTED_EDGE('',*,*,#3289,.T.);
#4340=ORIENTED_EDGE('',*,*,#3290,.F.);
#4341=ORIENTED_EDGE('',*,*,#3289,.F.);
#4342=ORIENTED_EDGE('',*,*,#3291,.F.);
#4343=ORIENTED_EDGE('',*,*,#3292,.T.);
#4344=ORIENTED_EDGE('',*,*,#3293,.F.);
#4345=ORIENTED_EDGE('',*,*,#3292,.F.);
#4346=ORIENTED_EDGE('',*,*,#3294,.F.);
#4347=ORIENTED_EDGE('',*,*,#3295,.T.);
#4348=ORIENTED_EDGE('',*,*,#3296,.T.);
#4349=ORIENTED_EDGE('',*,*,#3295,.F.);
#4350=ORIENTED_EDGE('',*,*,#3296,.F.);
#4351=ORIENTED_EDGE('',*,*,#3297,.F.);
#4352=ORIENTED_EDGE('',*,*,#3298,.F.);
#4353=ORIENTED_EDGE('',*,*,#3299,.T.);
#4354=ORIENTED_EDGE('',*,*,#3300,.T.);
#4355=ORIENTED_EDGE('',*,*,#3299,.F.);
#4356=ORIENTED_EDGE('',*,*,#3300,.F.);
#4357=ORIENTED_EDGE('',*,*,#3301,.F.);
#4358=ORIENTED_EDGE('',*,*,#3297,.T.);
#4359=ORIENTED_EDGE('',*,*,#3302,.T.);
#4360=ORIENTED_EDGE('',*,*,#3303,.F.);
#4361=ORIENTED_EDGE('',*,*,#3302,.F.);
#4362=ORIENTED_EDGE('',*,*,#3301,.T.);
#4363=ORIENTED_EDGE('',*,*,#3304,.T.);
#4364=ORIENTED_EDGE('',*,*,#3305,.F.);
#4365=ORIENTED_EDGE('',*,*,#3304,.F.);
#4366=ORIENTED_EDGE('',*,*,#3306,.F.);
#4367=ORIENTED_EDGE('',*,*,#3307,.F.);
#4368=ORIENTED_EDGE('',*,*,#3308,.F.);
#4369=ORIENTED_EDGE('',*,*,#3309,.T.);
#4370=ORIENTED_EDGE('',*,*,#3310,.F.);
#4371=ORIENTED_EDGE('',*,*,#3311,.T.);
#4372=ORIENTED_EDGE('',*,*,#3312,.F.);
#4373=ORIENTED_EDGE('',*,*,#3313,.F.);
#4374=ORIENTED_EDGE('',*,*,#3314,.F.);
#4375=ORIENTED_EDGE('',*,*,#3315,.T.);
#4376=ORIENTED_EDGE('',*,*,#3316,.F.);
#4377=ORIENTED_EDGE('',*,*,#3317,.F.);
#4378=ORIENTED_EDGE('',*,*,#3318,.F.);
#4379=ORIENTED_EDGE('',*,*,#3319,.T.);
#4380=ORIENTED_EDGE('',*,*,#3320,.F.);
#4381=ORIENTED_EDGE('',*,*,#3321,.F.);
#4382=ORIENTED_EDGE('',*,*,#3322,.F.);
#4383=ORIENTED_EDGE('',*,*,#3323,.T.);
#4384=ORIENTED_EDGE('',*,*,#3324,.F.);
#4385=ORIENTED_EDGE('',*,*,#3325,.F.);
#4386=ORIENTED_EDGE('',*,*,#3326,.F.);
#4387=ORIENTED_EDGE('',*,*,#3327,.F.);
#4388=ORIENTED_EDGE('',*,*,#3328,.F.);
#4389=ORIENTED_EDGE('',*,*,#3329,.T.);
#4390=ORIENTED_EDGE('',*,*,#3330,.F.);
#4391=ORIENTED_EDGE('',*,*,#3331,.F.);
#4392=ORIENTED_EDGE('',*,*,#3332,.F.);
#4393=ORIENTED_EDGE('',*,*,#3333,.T.);
#4394=ORIENTED_EDGE('',*,*,#3334,.F.);
#4395=ORIENTED_EDGE('',*,*,#3303,.T.);
#4396=ORIENTED_EDGE('',*,*,#3335,.F.);
#4397=ORIENTED_EDGE('',*,*,#3305,.T.);
#4398=ORIENTED_EDGE('',*,*,#3336,.F.);
#4399=ORIENTED_EDGE('',*,*,#3309,.F.);
#4400=ORIENTED_EDGE('',*,*,#3337,.F.);
#4401=ORIENTED_EDGE('',*,*,#3323,.F.);
#4402=ORIENTED_EDGE('',*,*,#3338,.F.);
#4403=ORIENTED_EDGE('',*,*,#3329,.F.);
#4404=ORIENTED_EDGE('',*,*,#3339,.F.);
#4405=ORIENTED_EDGE('',*,*,#3311,.F.);
#4406=ORIENTED_EDGE('',*,*,#3340,.F.);
#4407=ORIENTED_EDGE('',*,*,#3333,.F.);
#4408=ORIENTED_EDGE('',*,*,#3341,.F.);
#4409=ORIENTED_EDGE('',*,*,#3315,.F.);
#4410=ORIENTED_EDGE('',*,*,#3342,.F.);
#4411=ORIENTED_EDGE('',*,*,#3343,.F.);
#4412=ORIENTED_EDGE('',*,*,#3344,.F.);
#4413=ORIENTED_EDGE('',*,*,#3319,.F.);
#4414=ORIENTED_EDGE('',*,*,#3345,.F.);
#4415=ORIENTED_EDGE('',*,*,#3346,.F.);
#4416=ORIENTED_EDGE('',*,*,#3347,.F.);
#4417=ORIENTED_EDGE('',*,*,#3343,.T.);
#4418=ORIENTED_EDGE('',*,*,#3348,.T.);
#4419=ORIENTED_EDGE('',*,*,#3349,.F.);
#4420=ORIENTED_EDGE('',*,*,#3350,.F.);
#4421=ORIENTED_EDGE('',*,*,#3351,.F.);
#4422=ORIENTED_EDGE('',*,*,#3352,.F.);
#4423=ORIENTED_EDGE('',*,*,#3353,.F.);
#4424=ORIENTED_EDGE('',*,*,#3320,.T.);
#4425=ORIENTED_EDGE('',*,*,#3344,.T.);
#4426=ORIENTED_EDGE('',*,*,#3347,.T.);
#4427=ORIENTED_EDGE('',*,*,#3354,.T.);
#4428=ORIENTED_EDGE('',*,*,#3355,.F.);
#4429=ORIENTED_EDGE('',*,*,#3356,.F.);
#4430=ORIENTED_EDGE('',*,*,#3357,.F.);
#4431=ORIENTED_EDGE('',*,*,#3358,.F.);
#4432=ORIENTED_EDGE('',*,*,#3359,.F.);
#4433=ORIENTED_EDGE('',*,*,#3360,.T.);
#4434=ORIENTED_EDGE('',*,*,#3316,.T.);
#4435=ORIENTED_EDGE('',*,*,#3341,.T.);
#4436=ORIENTED_EDGE('',*,*,#3332,.T.);
#4437=ORIENTED_EDGE('',*,*,#3361,.T.);
#4438=ORIENTED_EDGE('',*,*,#3362,.F.);
#4439=ORIENTED_EDGE('',*,*,#3363,.F.);
#4440=ORIENTED_EDGE('',*,*,#3364,.F.);
#4441=ORIENTED_EDGE('',*,*,#3365,.F.);
#4442=ORIENTED_EDGE('',*,*,#3366,.F.);
#4443=ORIENTED_EDGE('',*,*,#3367,.T.);
#4444=ORIENTED_EDGE('',*,*,#3312,.T.);
#4445=ORIENTED_EDGE('',*,*,#3339,.T.);
#4446=ORIENTED_EDGE('',*,*,#3328,.T.);
#4447=ORIENTED_EDGE('',*,*,#3368,.T.);
#4448=ORIENTED_EDGE('',*,*,#3369,.F.);
#4449=ORIENTED_EDGE('',*,*,#3370,.F.);
#4450=ORIENTED_EDGE('',*,*,#3371,.F.);
#4451=ORIENTED_EDGE('',*,*,#3372,.F.);
#4452=ORIENTED_EDGE('',*,*,#3373,.F.);
#4453=ORIENTED_EDGE('',*,*,#3374,.T.);
#4454=ORIENTED_EDGE('',*,*,#3306,.T.);
#4455=ORIENTED_EDGE('',*,*,#3336,.T.);
#4456=ORIENTED_EDGE('',*,*,#3322,.T.);
#4457=ORIENTED_EDGE('',*,*,#3375,.F.);
#4458=ORIENTED_EDGE('',*,*,#3376,.T.);
#4459=ORIENTED_EDGE('',*,*,#3377,.T.);
#4460=ORIENTED_EDGE('',*,*,#3378,.T.);
#4461=ORIENTED_EDGE('',*,*,#3379,.F.);
#4462=ORIENTED_EDGE('',*,*,#3321,.T.);
#4463=ORIENTED_EDGE('',*,*,#3360,.F.);
#4464=ORIENTED_EDGE('',*,*,#3380,.T.);
#4465=ORIENTED_EDGE('',*,*,#3348,.F.);
#4466=ORIENTED_EDGE('',*,*,#3381,.T.);
#4467=ORIENTED_EDGE('',*,*,#3354,.F.);
#4468=ORIENTED_EDGE('',*,*,#3346,.T.);
#4469=ORIENTED_EDGE('',*,*,#3382,.F.);
#4470=ORIENTED_EDGE('',*,*,#3383,.T.);
#4471=ORIENTED_EDGE('',*,*,#3361,.F.);
#4472=ORIENTED_EDGE('',*,*,#3331,.T.);
#4473=ORIENTED_EDGE('',*,*,#3384,.F.);
#4474=ORIENTED_EDGE('',*,*,#3385,.T.);
#4475=ORIENTED_EDGE('',*,*,#3368,.F.);
#4476=ORIENTED_EDGE('',*,*,#3327,.T.);
#4477=ORIENTED_EDGE('',*,*,#3386,.F.);
#4478=ORIENTED_EDGE('',*,*,#3387,.T.);
#4479=ORIENTED_EDGE('',*,*,#3388,.T.);
#4480=ORIENTED_EDGE('',*,*,#3375,.T.);
#4481=ORIENTED_EDGE('',*,*,#3325,.T.);
#4482=ORIENTED_EDGE('',*,*,#3389,.T.);
#4483=ORIENTED_EDGE('',*,*,#3390,.F.);
#4484=ORIENTED_EDGE('',*,*,#3391,.T.);
#4485=ORIENTED_EDGE('',*,*,#3392,.F.);
#4486=ORIENTED_EDGE('',*,*,#3393,.T.);
#4487=ORIENTED_EDGE('',*,*,#3394,.F.);
#4488=ORIENTED_EDGE('',*,*,#3395,.T.);
#4489=ORIENTED_EDGE('',*,*,#3396,.F.);
#4490=ORIENTED_EDGE('',*,*,#3397,.T.);
#4491=ORIENTED_EDGE('',*,*,#3307,.T.);
#4492=ORIENTED_EDGE('',*,*,#3379,.T.);
#4493=ORIENTED_EDGE('',*,*,#3398,.T.);
#4494=ORIENTED_EDGE('',*,*,#3399,.T.);
#4495=ORIENTED_EDGE('',*,*,#3400,.F.);
#4496=ORIENTED_EDGE('',*,*,#3313,.T.);
#4497=ORIENTED_EDGE('',*,*,#3374,.F.);
#4498=ORIENTED_EDGE('',*,*,#3401,.T.);
#4499=ORIENTED_EDGE('',*,*,#3402,.F.);
#4500=ORIENTED_EDGE('',*,*,#3317,.T.);
#4501=ORIENTED_EDGE('',*,*,#3367,.F.);
#4502=ORIENTED_EDGE('',*,*,#3403,.T.);
#4503=ORIENTED_EDGE('',*,*,#3404,.F.);
#4504=ORIENTED_EDGE('',*,*,#3405,.T.);
#4505=ORIENTED_EDGE('',*,*,#3406,.T.);
#4506=ORIENTED_EDGE('',*,*,#3407,.T.);
#4507=ORIENTED_EDGE('',*,*,#3408,.T.);
#4508=ORIENTED_EDGE('',*,*,#3409,.T.);
#4509=ORIENTED_EDGE('',*,*,#3410,.F.);
#4510=ORIENTED_EDGE('',*,*,#3411,.F.);
#4511=ORIENTED_EDGE('',*,*,#3412,.T.);
#4512=ORIENTED_EDGE('',*,*,#3335,.T.);
#4513=ORIENTED_EDGE('',*,*,#3412,.F.);
#4514=ORIENTED_EDGE('',*,*,#3413,.F.);
#4515=ORIENTED_EDGE('',*,*,#3414,.T.);
#4516=ORIENTED_EDGE('',*,*,#3334,.T.);
#4517=ORIENTED_EDGE('',*,*,#3414,.F.);
#4518=ORIENTED_EDGE('',*,*,#3415,.F.);
#4519=ORIENTED_EDGE('',*,*,#3410,.T.);
#4520=ORIENTED_EDGE('',*,*,#3416,.F.);
#4521=ORIENTED_EDGE('',*,*,#3417,.F.);
#4522=ORIENTED_EDGE('',*,*,#3418,.F.);
#4523=ORIENTED_EDGE('',*,*,#3419,.F.);
#4524=ORIENTED_EDGE('',*,*,#3349,.T.);
#4525=ORIENTED_EDGE('',*,*,#3380,.F.);
#4526=ORIENTED_EDGE('',*,*,#3359,.T.);
#4527=ORIENTED_EDGE('',*,*,#3420,.T.);
#4528=ORIENTED_EDGE('',*,*,#3415,.T.);
#4529=ORIENTED_EDGE('',*,*,#3421,.T.);
#4530=ORIENTED_EDGE('',*,*,#3422,.T.);
#4531=ORIENTED_EDGE('',*,*,#3405,.F.);
#4532=ORIENTED_EDGE('',*,*,#3350,.T.);
#4533=ORIENTED_EDGE('',*,*,#3420,.F.);
#4534=ORIENTED_EDGE('',*,*,#3358,.T.);
#4535=ORIENTED_EDGE('',*,*,#3423,.F.);
#4536=ORIENTED_EDGE('',*,*,#3419,.T.);
#4537=ORIENTED_EDGE('',*,*,#3424,.F.);
#4538=ORIENTED_EDGE('',*,*,#3425,.F.);
#4539=ORIENTED_EDGE('',*,*,#3421,.F.);
#4540=ORIENTED_EDGE('',*,*,#3351,.T.);
#4541=ORIENTED_EDGE('',*,*,#3423,.T.);
#4542=ORIENTED_EDGE('',*,*,#3357,.T.);
#4543=ORIENTED_EDGE('',*,*,#3426,.T.);
#4544=ORIENTED_EDGE('',*,*,#3284,.T.);
#4545=ORIENTED_EDGE('',*,*,#3293,.T.);
#4546=ORIENTED_EDGE('',*,*,#3411,.T.);
#4547=ORIENTED_EDGE('',*,*,#3418,.T.);
#4548=ORIENTED_EDGE('',*,*,#3427,.T.);
#4549=ORIENTED_EDGE('',*,*,#3428,.T.);
#4550=ORIENTED_EDGE('',*,*,#3424,.T.);
#4551=ORIENTED_EDGE('',*,*,#3352,.T.);
#4552=ORIENTED_EDGE('',*,*,#3426,.F.);
#4553=ORIENTED_EDGE('',*,*,#3356,.T.);
#4554=ORIENTED_EDGE('',*,*,#3429,.F.);
#4555=ORIENTED_EDGE('',*,*,#3353,.T.);
#4556=ORIENTED_EDGE('',*,*,#3429,.T.);
#4557=ORIENTED_EDGE('',*,*,#3355,.T.);
#4558=ORIENTED_EDGE('',*,*,#3381,.F.);
#4559=ORIENTED_EDGE('',*,*,#3416,.T.);
#4560=ORIENTED_EDGE('',*,*,#3409,.F.);
#4561=ORIENTED_EDGE('',*,*,#3430,.T.);
#4562=ORIENTED_EDGE('',*,*,#3431,.T.);
#4563=ORIENTED_EDGE('',*,*,#3318,.T.);
#4564=ORIENTED_EDGE('',*,*,#3404,.T.);
#4565=ORIENTED_EDGE('',*,*,#3432,.F.);
#4566=ORIENTED_EDGE('',*,*,#3433,.F.);
#4567=ORIENTED_EDGE('',*,*,#3434,.F.);
#4568=ORIENTED_EDGE('',*,*,#3435,.F.);
#4569=ORIENTED_EDGE('',*,*,#3436,.F.);
#4570=ORIENTED_EDGE('',*,*,#3382,.T.);
#4571=ORIENTED_EDGE('',*,*,#3345,.T.);
#4572=ORIENTED_EDGE('',*,*,#3342,.T.);
#4573=ORIENTED_EDGE('',*,*,#3432,.T.);
#4574=ORIENTED_EDGE('',*,*,#3403,.F.);
#4575=ORIENTED_EDGE('',*,*,#3366,.T.);
#4576=ORIENTED_EDGE('',*,*,#3437,.T.);
#4577=ORIENTED_EDGE('',*,*,#3433,.T.);
#4578=ORIENTED_EDGE('',*,*,#3437,.F.);
#4579=ORIENTED_EDGE('',*,*,#3365,.T.);
#4580=ORIENTED_EDGE('',*,*,#3438,.F.);
#4581=ORIENTED_EDGE('',*,*,#3434,.T.);
#4582=ORIENTED_EDGE('',*,*,#3438,.T.);
#4583=ORIENTED_EDGE('',*,*,#3364,.T.);
#4584=ORIENTED_EDGE('',*,*,#3439,.T.);
#4585=ORIENTED_EDGE('',*,*,#3435,.T.);
#4586=ORIENTED_EDGE('',*,*,#3439,.F.);
#4587=ORIENTED_EDGE('',*,*,#3363,.T.);
#4588=ORIENTED_EDGE('',*,*,#3440,.F.);
#4589=ORIENTED_EDGE('',*,*,#3436,.T.);
#4590=ORIENTED_EDGE('',*,*,#3440,.T.);
#4591=ORIENTED_EDGE('',*,*,#3362,.T.);
#4592=ORIENTED_EDGE('',*,*,#3383,.F.);
#4593=ORIENTED_EDGE('',*,*,#3314,.T.);
#4594=ORIENTED_EDGE('',*,*,#3402,.T.);
#4595=ORIENTED_EDGE('',*,*,#3441,.F.);
#4596=ORIENTED_EDGE('',*,*,#3442,.F.);
#4597=ORIENTED_EDGE('',*,*,#3443,.F.);
#4598=ORIENTED_EDGE('',*,*,#3444,.F.);
#4599=ORIENTED_EDGE('',*,*,#3445,.F.);
#4600=ORIENTED_EDGE('',*,*,#3384,.T.);
#4601=ORIENTED_EDGE('',*,*,#3330,.T.);
#4602=ORIENTED_EDGE('',*,*,#3340,.T.);
#4603=ORIENTED_EDGE('',*,*,#3441,.T.);
#4604=ORIENTED_EDGE('',*,*,#3401,.F.);
#4605=ORIENTED_EDGE('',*,*,#3373,.T.);
#4606=ORIENTED_EDGE('',*,*,#3446,.T.);
#4607=ORIENTED_EDGE('',*,*,#3442,.T.);
#4608=ORIENTED_EDGE('',*,*,#3446,.F.);
#4609=ORIENTED_EDGE('',*,*,#3372,.T.);
#4610=ORIENTED_EDGE('',*,*,#3447,.F.);
#4611=ORIENTED_EDGE('',*,*,#3443,.T.);
#4612=ORIENTED_EDGE('',*,*,#3447,.T.);
#4613=ORIENTED_EDGE('',*,*,#3371,.T.);
#4614=ORIENTED_EDGE('',*,*,#3448,.T.);
#4615=ORIENTED_EDGE('',*,*,#3287,.T.);
#4616=ORIENTED_EDGE('',*,*,#3290,.T.);
#4617=ORIENTED_EDGE('',*,*,#3413,.T.);
#4618=ORIENTED_EDGE('',*,*,#3444,.T.);
#4619=ORIENTED_EDGE('',*,*,#3448,.F.);
#4620=ORIENTED_EDGE('',*,*,#3370,.T.);
#4621=ORIENTED_EDGE('',*,*,#3449,.F.);
#4622=ORIENTED_EDGE('',*,*,#3445,.T.);
#4623=ORIENTED_EDGE('',*,*,#3449,.T.);
#4624=ORIENTED_EDGE('',*,*,#3369,.T.);
#4625=ORIENTED_EDGE('',*,*,#3385,.F.);
#4626=ORIENTED_EDGE('',*,*,#3310,.T.);
#4627=ORIENTED_EDGE('',*,*,#3400,.T.);
#4628=ORIENTED_EDGE('',*,*,#3450,.F.);
#4629=ORIENTED_EDGE('',*,*,#3451,.F.);
#4630=ORIENTED_EDGE('',*,*,#3452,.F.);
#4631=ORIENTED_EDGE('',*,*,#3453,.F.);
#4632=ORIENTED_EDGE('',*,*,#3454,.F.);
#4633=ORIENTED_EDGE('',*,*,#3386,.T.);
#4634=ORIENTED_EDGE('',*,*,#3326,.T.);
#4635=ORIENTED_EDGE('',*,*,#3338,.T.);
#4636=ORIENTED_EDGE('',*,*,#3450,.T.);
#4637=ORIENTED_EDGE('',*,*,#3399,.F.);
#4638=ORIENTED_EDGE('',*,*,#3455,.T.);
#4639=ORIENTED_EDGE('',*,*,#3456,.T.);
#4640=ORIENTED_EDGE('',*,*,#3451,.T.);
#4641=ORIENTED_EDGE('',*,*,#3456,.F.);
#4642=ORIENTED_EDGE('',*,*,#3457,.F.);
#4643=ORIENTED_EDGE('',*,*,#3458,.F.);
#4644=ORIENTED_EDGE('',*,*,#3452,.T.);
#4645=ORIENTED_EDGE('',*,*,#3458,.T.);
#4646=ORIENTED_EDGE('',*,*,#3459,.T.);
#4647=ORIENTED_EDGE('',*,*,#3460,.T.);
#4648=ORIENTED_EDGE('',*,*,#3454,.T.);
#4649=ORIENTED_EDGE('',*,*,#3461,.T.);
#4650=ORIENTED_EDGE('',*,*,#3462,.T.);
#4651=ORIENTED_EDGE('',*,*,#3387,.F.);
#4652=ORIENTED_EDGE('',*,*,#3453,.T.);
#4653=ORIENTED_EDGE('',*,*,#3460,.F.);
#4654=ORIENTED_EDGE('',*,*,#3463,.F.);
#4655=ORIENTED_EDGE('',*,*,#3461,.F.);
#4656=ORIENTED_EDGE('',*,*,#3464,.T.);
#4657=ORIENTED_EDGE('',*,*,#3465,.T.);
#4658=ORIENTED_EDGE('',*,*,#3463,.T.);
#4659=ORIENTED_EDGE('',*,*,#3466,.T.);
#4660=ORIENTED_EDGE('',*,*,#3467,.T.);
#4661=ORIENTED_EDGE('',*,*,#3468,.T.);
#4662=ORIENTED_EDGE('',*,*,#3457,.T.);
#4663=ORIENTED_EDGE('',*,*,#3469,.T.);
#4664=ORIENTED_EDGE('',*,*,#3470,.T.);
#4665=ORIENTED_EDGE('',*,*,#3464,.F.);
#4666=ORIENTED_EDGE('',*,*,#3459,.F.);
#4667=ORIENTED_EDGE('',*,*,#3470,.F.);
#4668=ORIENTED_EDGE('',*,*,#3377,.F.);
#4669=ORIENTED_EDGE('',*,*,#3398,.F.);
#4670=ORIENTED_EDGE('',*,*,#3378,.F.);
#4671=ORIENTED_EDGE('',*,*,#3469,.F.);
#4672=ORIENTED_EDGE('',*,*,#3455,.F.);
#4673=ORIENTED_EDGE('',*,*,#3471,.T.);
#4674=ORIENTED_EDGE('',*,*,#3425,.T.);
#4675=ORIENTED_EDGE('',*,*,#3472,.T.);
#4676=ORIENTED_EDGE('',*,*,#3472,.F.);
#4677=ORIENTED_EDGE('',*,*,#3428,.F.);
#4678=ORIENTED_EDGE('',*,*,#3468,.F.);
#4679=ORIENTED_EDGE('',*,*,#3473,.F.);
#4680=ORIENTED_EDGE('',*,*,#3406,.F.);
#4681=ORIENTED_EDGE('',*,*,#3422,.F.);
#4682=ORIENTED_EDGE('',*,*,#3471,.F.);
#4683=ORIENTED_EDGE('',*,*,#3474,.F.);
#4684=ORIENTED_EDGE('',*,*,#3408,.F.);
#4685=ORIENTED_EDGE('',*,*,#3475,.F.);
#4686=ORIENTED_EDGE('',*,*,#3467,.F.);
#4687=ORIENTED_EDGE('',*,*,#3430,.F.);
#4688=ORIENTED_EDGE('',*,*,#3417,.T.);
#4689=ORIENTED_EDGE('',*,*,#3431,.F.);
#4690=ORIENTED_EDGE('',*,*,#3466,.F.);
#4691=ORIENTED_EDGE('',*,*,#3427,.F.);
#4692=ORIENTED_EDGE('',*,*,#3388,.F.);
#4693=ORIENTED_EDGE('',*,*,#3462,.F.);
#4694=ORIENTED_EDGE('',*,*,#3465,.F.);
#4695=ORIENTED_EDGE('',*,*,#3376,.F.);
#4696=ORIENTED_EDGE('',*,*,#3474,.T.);
#4697=ORIENTED_EDGE('',*,*,#3473,.T.);
#4698=ORIENTED_EDGE('',*,*,#3475,.T.);
#4699=ORIENTED_EDGE('',*,*,#3407,.F.);
#4700=ORIENTED_EDGE('',*,*,#3476,.F.);
#4701=ORIENTED_EDGE('',*,*,#3477,.F.);
#4702=ORIENTED_EDGE('',*,*,#3478,.F.);
#4703=ORIENTED_EDGE('',*,*,#3479,.F.);
#4704=ORIENTED_EDGE('',*,*,#3480,.F.);
#4705=ORIENTED_EDGE('',*,*,#3481,.F.);
#4706=ORIENTED_EDGE('',*,*,#3482,.F.);
#4707=ORIENTED_EDGE('',*,*,#3483,.F.);
#4708=ORIENTED_EDGE('',*,*,#3484,.F.);
#4709=ORIENTED_EDGE('',*,*,#3476,.T.);
#4710=ORIENTED_EDGE('',*,*,#3485,.T.);
#4711=ORIENTED_EDGE('',*,*,#3483,.T.);
#4712=ORIENTED_EDGE('',*,*,#3486,.T.);
#4713=ORIENTED_EDGE('',*,*,#3396,.T.);
#4714=ORIENTED_EDGE('',*,*,#3487,.T.);
#4715=ORIENTED_EDGE('',*,*,#3484,.T.);
#4716=ORIENTED_EDGE('',*,*,#3488,.T.);
#4717=ORIENTED_EDGE('',*,*,#3489,.F.);
#4718=ORIENTED_EDGE('',*,*,#3490,.F.);
#4719=ORIENTED_EDGE('',*,*,#3491,.F.);
#4720=ORIENTED_EDGE('',*,*,#3490,.T.);
#4721=ORIENTED_EDGE('',*,*,#3492,.T.);
#4722=ORIENTED_EDGE('',*,*,#3480,.T.);
#4723=ORIENTED_EDGE('',*,*,#3493,.T.);
#4724=ORIENTED_EDGE('',*,*,#3482,.T.);
#4725=ORIENTED_EDGE('',*,*,#3494,.T.);
#4726=ORIENTED_EDGE('',*,*,#3491,.T.);
#4727=ORIENTED_EDGE('',*,*,#3495,.T.);
#4728=ORIENTED_EDGE('',*,*,#3394,.T.);
#4729=ORIENTED_EDGE('',*,*,#3496,.T.);
#4730=ORIENTED_EDGE('',*,*,#3489,.T.);
#4731=ORIENTED_EDGE('',*,*,#3497,.T.);
#4732=ORIENTED_EDGE('',*,*,#3392,.T.);
#4733=ORIENTED_EDGE('',*,*,#3498,.T.);
#4734=ORIENTED_EDGE('',*,*,#3481,.T.);
#4735=ORIENTED_EDGE('',*,*,#3499,.T.);
#4736=ORIENTED_EDGE('',*,*,#3479,.T.);
#4737=ORIENTED_EDGE('',*,*,#3500,.T.);
#4738=ORIENTED_EDGE('',*,*,#3477,.T.);
#4739=ORIENTED_EDGE('',*,*,#3501,.T.);
#4740=ORIENTED_EDGE('',*,*,#3390,.T.);
#4741=ORIENTED_EDGE('',*,*,#3502,.T.);
#4742=ORIENTED_EDGE('',*,*,#3478,.T.);
#4743=ORIENTED_EDGE('',*,*,#3503,.T.);
#4744=ORIENTED_EDGE('',*,*,#3497,.F.);
#4745=ORIENTED_EDGE('',*,*,#3494,.F.);
#4746=ORIENTED_EDGE('',*,*,#3487,.F.);
#4747=ORIENTED_EDGE('',*,*,#3395,.F.);
#4748=ORIENTED_EDGE('',*,*,#3308,.T.);
#4749=ORIENTED_EDGE('',*,*,#3397,.F.);
#4750=ORIENTED_EDGE('',*,*,#3488,.F.);
#4751=ORIENTED_EDGE('',*,*,#3485,.F.);
#4752=ORIENTED_EDGE('',*,*,#3502,.F.);
#4753=ORIENTED_EDGE('',*,*,#3389,.F.);
#4754=ORIENTED_EDGE('',*,*,#3324,.T.);
#4755=ORIENTED_EDGE('',*,*,#3337,.T.);
#4756=ORIENTED_EDGE('',*,*,#3493,.F.);
#4757=ORIENTED_EDGE('',*,*,#3501,.F.);
#4758=ORIENTED_EDGE('',*,*,#3486,.F.);
#4759=ORIENTED_EDGE('',*,*,#3495,.F.);
#4760=ORIENTED_EDGE('',*,*,#3298,.T.);
#4761=ORIENTED_EDGE('',*,*,#3294,.T.);
#4762=ORIENTED_EDGE('',*,*,#3291,.T.);
#4763=ORIENTED_EDGE('',*,*,#3288,.T.);
#4764=ORIENTED_EDGE('',*,*,#3285,.T.);
#4765=ORIENTED_EDGE('',*,*,#3282,.T.);
#4766=ORIENTED_EDGE('',*,*,#3498,.F.);
#4767=ORIENTED_EDGE('',*,*,#3391,.F.);
#4768=ORIENTED_EDGE('',*,*,#3503,.F.);
#4769=ORIENTED_EDGE('',*,*,#3500,.F.);
#4770=ORIENTED_EDGE('',*,*,#3496,.F.);
#4771=ORIENTED_EDGE('',*,*,#3393,.F.);
#4772=ORIENTED_EDGE('',*,*,#3499,.F.);
#4773=ORIENTED_EDGE('',*,*,#3492,.F.);
#5998=CYLINDRICAL_SURFACE('',#6687,0.15);
#5999=CYLINDRICAL_SURFACE('',#6690,0.15);
#6000=CYLINDRICAL_SURFACE('',#6693,0.15);
#6001=CYLINDRICAL_SURFACE('',#6696,0.15);
#6002=CYLINDRICAL_SURFACE('',#6699,0.3);
#6003=CYLINDRICAL_SURFACE('',#6704,0.3);
#6004=CYLINDRICAL_SURFACE('',#6709,0.17);
#6005=CYLINDRICAL_SURFACE('',#6711,0.17);
#6006=CYLINDRICAL_SURFACE('',#6735,0.4);
#6007=CYLINDRICAL_SURFACE('',#6737,0.4);
#6008=CYLINDRICAL_SURFACE('',#6761,0.1);
#6009=CYLINDRICAL_SURFACE('',#6765,0.1);
#6010=CYLINDRICAL_SURFACE('',#6779,0.3);
#6011=CYLINDRICAL_SURFACE('',#6784,0.3);
#6160=ADVANCED_FACE('',(#829),#5998,.F.);
#6161=ADVANCED_FACE('',(#830),#5999,.F.);
#6162=ADVANCED_FACE('',(#831),#6000,.F.);
#6163=ADVANCED_FACE('',(#832),#6001,.F.);
#6164=ADVANCED_FACE('',(#833),#6002,.F.);
#6165=ADVANCED_FACE('',(#834,#586),#668,.F.);
#6166=ADVANCED_FACE('',(#835),#6003,.F.);
#6167=ADVANCED_FACE('',(#836,#587),#669,.F.);
#6168=ADVANCED_FACE('',(#837),#6004,.F.);
#6169=ADVANCED_FACE('',(#838),#6005,.F.);
#6170=ADVANCED_FACE('',(#839),#670,.F.);
#6171=ADVANCED_FACE('',(#840),#671,.F.);
#6172=ADVANCED_FACE('',(#841),#672,.F.);
#6173=ADVANCED_FACE('',(#842),#673,.F.);
#6174=ADVANCED_FACE('',(#843),#674,.F.);
#6175=ADVANCED_FACE('',(#844),#675,.F.);
#6176=ADVANCED_FACE('',(#845),#676,.F.);
#6177=ADVANCED_FACE('',(#846,#588),#677,.F.);
#6178=ADVANCED_FACE('',(#847,#589),#678,.F.);
#6179=ADVANCED_FACE('',(#848),#679,.F.);
#6180=ADVANCED_FACE('',(#849),#680,.F.);
#6181=ADVANCED_FACE('',(#850),#681,.F.);
#6182=ADVANCED_FACE('',(#851),#682,.F.);
#6183=ADVANCED_FACE('',(#852),#683,.F.);
#6184=ADVANCED_FACE('',(#853),#684,.T.);
#6185=ADVANCED_FACE('',(#854),#685,.T.);
#6186=ADVANCED_FACE('',(#855),#686,.T.);
#6187=ADVANCED_FACE('',(#856),#687,.T.);
#6188=ADVANCED_FACE('',(#857),#688,.T.);
#6189=ADVANCED_FACE('',(#858,#590),#689,.F.);
#6190=ADVANCED_FACE('',(#859),#6006,.T.);
#6191=ADVANCED_FACE('',(#860),#6007,.T.);
#6192=ADVANCED_FACE('',(#861),#690,.T.);
#6193=ADVANCED_FACE('',(#862),#91,.T.);
#6194=ADVANCED_FACE('',(#863),#92,.T.);
#6195=ADVANCED_FACE('',(#864),#93,.T.);
#6196=ADVANCED_FACE('',(#865),#94,.T.);
#6197=ADVANCED_FACE('',(#866,#591,#592,#593),#691,.F.);
#6198=ADVANCED_FACE('',(#867),#692,.F.);
#6199=ADVANCED_FACE('',(#868),#95,.T.);
#6200=ADVANCED_FACE('',(#869),#96,.T.);
#6201=ADVANCED_FACE('',(#870),#97,.T.);
#6202=ADVANCED_FACE('',(#871),#693,.T.);
#6203=ADVANCED_FACE('',(#872),#98,.T.);
#6204=ADVANCED_FACE('',(#873),#99,.T.);
#6205=ADVANCED_FACE('',(#874),#694,.F.);
#6206=ADVANCED_FACE('',(#875),#100,.T.);
#6207=ADVANCED_FACE('',(#876),#101,.T.);
#6208=ADVANCED_FACE('',(#877),#695,.T.);
#6209=ADVANCED_FACE('',(#878),#102,.T.);
#6210=ADVANCED_FACE('',(#879),#103,.T.);
#6211=ADVANCED_FACE('',(#880,#594,#595,#596),#696,.F.);
#6212=ADVANCED_FACE('',(#881),#104,.T.);
#6213=ADVANCED_FACE('',(#882),#105,.T.);
#6214=ADVANCED_FACE('',(#883),#697,.T.);
#6215=ADVANCED_FACE('',(#884),#106,.T.);
#6216=ADVANCED_FACE('',(#885),#107,.T.);
#6217=ADVANCED_FACE('',(#886),#698,.F.);
#6218=ADVANCED_FACE('',(#887),#108,.T.);
#6219=ADVANCED_FACE('',(#888),#109,.T.);
#6220=ADVANCED_FACE('',(#889),#75,.F.);
#6221=ADVANCED_FACE('',(#890),#76,.F.);
#6222=ADVANCED_FACE('',(#891),#77,.F.);
#6223=ADVANCED_FACE('',(#892),#6008,.F.);
#6224=ADVANCED_FACE('',(#893),#110,.T.);
#6225=ADVANCED_FACE('',(#894),#78,.F.);
#6226=ADVANCED_FACE('',(#895),#6009,.F.);
#6227=ADVANCED_FACE('',(#896),#111,.T.);
#6228=ADVANCED_FACE('',(#897),#112,.T.);
#6229=ADVANCED_FACE('',(#898),#113,.T.);
#6230=ADVANCED_FACE('',(#899),#114,.T.);
#6231=ADVANCED_FACE('',(#900),#699,.T.);
#6232=ADVANCED_FACE('',(#901),#79,.T.);
#6233=ADVANCED_FACE('',(#902),#80,.T.);
#6234=ADVANCED_FACE('',(#903),#81,.T.);
#6235=ADVANCED_FACE('',(#904),#6010,.T.);
#6236=ADVANCED_FACE('',(#905),#115,.F.);
#6237=ADVANCED_FACE('',(#906),#82,.T.);
#6238=ADVANCED_FACE('',(#907),#6011,.T.);
#6239=ADVANCED_FACE('',(#908),#116,.F.);
#6240=ADVANCED_FACE('',(#909),#117,.F.);
#6241=ADVANCED_FACE('',(#910),#118,.F.);
#6242=ADVANCED_FACE('',(#911),#119,.F.);
#6243=ADVANCED_FACE('',(#912),#120,.F.);
#6244=ADVANCED_FACE('',(#913),#121,.F.);
#6245=ADVANCED_FACE('',(#914),#700,.F.);
#6246=ADVANCED_FACE('',(#915,#597,#598,#599,#600,#601,#602),#701,.T.);
#6247=ADVANCED_FACE('',(#916),#122,.F.);
#6248=ADVANCED_FACE('',(#917),#702,.F.);
#6489=CLOSED_SHELL('',(#6160,#6161,#6162,#6163,#6164,#6165,#6166,#6167,
#6168,#6169,#6170,#6171,#6172,#6173,#6174,#6175,#6176,#6177,#6178,#6179,
#6180,#6181,#6182,#6183,#6184,#6185,#6186,#6187,#6188,#6189,#6190,#6191,
#6192,#6193,#6194,#6195,#6196,#6197,#6198,#6199,#6200,#6201,#6202,#6203,
#6204,#6205,#6206,#6207,#6208,#6209,#6210,#6211,#6212,#6213,#6214,#6215,
#6216,#6217,#6218,#6219,#6220,#6221,#6222,#6223,#6224,#6225,#6226,#6227,
#6228,#6229,#6230,#6231,#6232,#6233,#6234,#6235,#6236,#6237,#6238,#6239,
#6240,#6241,#6242,#6243,#6244,#6245,#6246,#6247,#6248));
#6686=AXIS2_PLACEMENT_3D('',#8696,#7336,#7337);
#6687=AXIS2_PLACEMENT_3D('',#8697,#7338,#7339);
#6688=AXIS2_PLACEMENT_3D('',#8699,#7340,#7341);
#6689=AXIS2_PLACEMENT_3D('',#8702,#7343,#7344);
#6690=AXIS2_PLACEMENT_3D('',#8703,#7345,#7346);
#6691=AXIS2_PLACEMENT_3D('',#8705,#7347,#7348);
#6692=AXIS2_PLACEMENT_3D('',#8708,#7350,#7351);
#6693=AXIS2_PLACEMENT_3D('',#8709,#7352,#7353);
#6694=AXIS2_PLACEMENT_3D('',#8711,#7354,#7355);
#6695=AXIS2_PLACEMENT_3D('',#8714,#7357,#7358);
#6696=AXIS2_PLACEMENT_3D('',#8715,#7359,#7360);
#6697=AXIS2_PLACEMENT_3D('',#8717,#7361,#7362);
#6698=AXIS2_PLACEMENT_3D('',#8720,#7364,#7365);
#6699=AXIS2_PLACEMENT_3D('',#8721,#7366,#7367);
#6700=AXIS2_PLACEMENT_3D('',#8723,#7368,#7369);
#6701=AXIS2_PLACEMENT_3D('',#8726,#7371,#7372);
#6702=AXIS2_PLACEMENT_3D('',#8727,#7373,#7374);
#6703=AXIS2_PLACEMENT_3D('',#8729,#7375,#7376);
#6704=AXIS2_PLACEMENT_3D('',#8730,#7377,#7378);
#6705=AXIS2_PLACEMENT_3D('',#8732,#7379,#7380);
#6706=AXIS2_PLACEMENT_3D('',#8735,#7382,#7383);
#6707=AXIS2_PLACEMENT_3D('',#8736,#7384,#7385);
#6708=AXIS2_PLACEMENT_3D('',#8738,#7386,#7387);
#6709=AXIS2_PLACEMENT_3D('',#8739,#7388,#7389);
#6710=AXIS2_PLACEMENT_3D('',#8742,#7391,#7392);
#6711=AXIS2_PLACEMENT_3D('',#8743,#7393,#7394);
#6712=AXIS2_PLACEMENT_3D('',#8746,#7396,#7397);
#6713=AXIS2_PLACEMENT_3D('',#8747,#7398,#7399);
#6714=AXIS2_PLACEMENT_3D('',#8756,#7404,#7405);
#6715=AXIS2_PLACEMENT_3D('',#8765,#7410,#7411);
#6716=AXIS2_PLACEMENT_3D('',#8774,#7416,#7417);
#6717=AXIS2_PLACEMENT_3D('',#8783,#7422,#7423);
#6718=AXIS2_PLACEMENT_3D('',#8792,#7428,#7429);
#6719=AXIS2_PLACEMENT_3D('',#8801,#7434,#7435);
#6720=AXIS2_PLACEMENT_3D('',#8810,#7440,#7441);
#6721=AXIS2_PLACEMENT_3D('',#8812,#7442,#7443);
#6722=AXIS2_PLACEMENT_3D('',#8813,#7444,#7445);
#6723=AXIS2_PLACEMENT_3D('',#8815,#7446,#7447);
#6724=AXIS2_PLACEMENT_3D('',#8816,#7448,#7449);
#6725=AXIS2_PLACEMENT_3D('',#8819,#7452,#7453);
#6726=AXIS2_PLACEMENT_3D('',#8822,#7456,#7457);
#6727=AXIS2_PLACEMENT_3D('',#8825,#7460,#7461);
#6728=AXIS2_PLACEMENT_3D('',#8831,#7465,#7466);
#6729=AXIS2_PLACEMENT_3D('',#8837,#7470,#7471);
#6730=AXIS2_PLACEMENT_3D('',#8914,#7474,#7475);
#6731=AXIS2_PLACEMENT_3D('',#8992,#7479,#7480);
#6732=AXIS2_PLACEMENT_3D('',#9070,#7484,#7485);
#6733=AXIS2_PLACEMENT_3D('',#9148,#7489,#7490);
#6734=AXIS2_PLACEMENT_3D('',#9164,#7494,#7495);
#6735=AXIS2_PLACEMENT_3D('',#9488,#7507,#7508);
#6736=AXIS2_PLACEMENT_3D('',#9490,#7509,#7510);
#6737=AXIS2_PLACEMENT_3D('',#9492,#7512,#7513);
#6738=AXIS2_PLACEMENT_3D('',#9494,#7514,#7515);
#6739=AXIS2_PLACEMENT_3D('',#9496,#7517,#7518);
#6740=AXIS2_PLACEMENT_3D('',#9664,#7520,#7521);
#6741=AXIS2_PLACEMENT_3D('',#9665,#7522,#7523);
#6742=AXIS2_PLACEMENT_3D('',#9670,#7524,#7525);
#6743=AXIS2_PLACEMENT_3D('',#9742,#7527,#7528);
#6744=AXIS2_PLACEMENT_3D('',#9860,#7530,#7531);
#6745=AXIS2_PLACEMENT_3D('',#9905,#7532,#7533);
#6746=AXIS2_PLACEMENT_3D('',#10023,#7535,#7536);
#6747=AXIS2_PLACEMENT_3D('',#10068,#7537,#7538);
#6748=AXIS2_PLACEMENT_3D('',#10188,#7540,#7541);
#6749=AXIS2_PLACEMENT_3D('',#10193,#7542,#7543);
#6750=AXIS2_PLACEMENT_3D('',#10245,#7545,#7546);
#6751=AXIS2_PLACEMENT_3D('',#10246,#7547,#7548);
#6752=AXIS2_PLACEMENT_3D('',#10247,#7549,#7550);
#6753=AXIS2_PLACEMENT_3D('',#10248,#7551,#7552);
#6754=AXIS2_PLACEMENT_3D('',#10249,#7553,#7554);
#6755=AXIS2_PLACEMENT_3D('',#10250,#7555,#7556);
#6756=AXIS2_PLACEMENT_3D('',#10252,#7557,#7558);
#6757=AXIS2_PLACEMENT_3D('',#10253,#7559,#7560);
#6758=AXIS2_PLACEMENT_3D('',#10254,#7561,#7562);
#6759=AXIS2_PLACEMENT_3D('',#10255,#7563,#7564);
#6760=AXIS2_PLACEMENT_3D('',#10256,#7565,#7566);
#6761=AXIS2_PLACEMENT_3D('',#10257,#7567,#7568);
#6762=AXIS2_PLACEMENT_3D('',#10278,#7569,#7570);
#6763=AXIS2_PLACEMENT_3D('',#10280,#7571,#7572);
#6764=AXIS2_PLACEMENT_3D('',#10281,#7573,#7574);
#6765=AXIS2_PLACEMENT_3D('',#10282,#7575,#7576);
#6766=AXIS2_PLACEMENT_3D('',#10372,#7578,#7579);
#6767=AXIS2_PLACEMENT_3D('',#10373,#7580,#7581);
#6768=AXIS2_PLACEMENT_3D('',#10376,#7582,#7583);
#6769=AXIS2_PLACEMENT_3D('',#10378,#7584,#7585);
#6770=AXIS2_PLACEMENT_3D('',#10379,#7586,#7587);
#6771=AXIS2_PLACEMENT_3D('',#10380,#7588,#7589);
#6772=AXIS2_PLACEMENT_3D('',#10383,#7590,#7591);
#6773=AXIS2_PLACEMENT_3D('',#10385,#7592,#7593);
#6774=AXIS2_PLACEMENT_3D('',#10386,#7594,#7595);
#6775=AXIS2_PLACEMENT_3D('',#10387,#7596,#7597);
#6776=AXIS2_PLACEMENT_3D('',#10390,#7598,#7599);
#6777=AXIS2_PLACEMENT_3D('',#10392,#7600,#7601);
#6778=AXIS2_PLACEMENT_3D('',#10393,#7602,#7603);
#6779=AXIS2_PLACEMENT_3D('',#10394,#7604,#7605);
#6780=AXIS2_PLACEMENT_3D('',#10425,#7608,#7609);
#6781=AXIS2_PLACEMENT_3D('',#10428,#7610,#7611);
#6782=AXIS2_PLACEMENT_3D('',#10430,#7612,#7613);
#6783=AXIS2_PLACEMENT_3D('',#10431,#7614,#7615);
#6784=AXIS2_PLACEMENT_3D('',#10432,#7616,#7617);
#6785=AXIS2_PLACEMENT_3D('',#10612,#7620,#7621);
#6786=AXIS2_PLACEMENT_3D('',#10613,#7622,#7623);
#6787=AXIS2_PLACEMENT_3D('',#10630,#7624,#7625);
#7336=DIRECTION('axis',(0.,0.,1.));
#7337=DIRECTION('refdir',(1.,0.,0.));
#7338=DIRECTION('center_axis',(0.,0.,-1.));
#7339=DIRECTION('ref_axis',(1.,0.,0.));
#7340=DIRECTION('center_axis',(1.01338750660366E-31,-1.26069923670246E-19,
-1.));
#7341=DIRECTION('ref_axis',(1.,0.,0.));
#7342=DIRECTION('',(0.,0.,-1.));
#7343=DIRECTION('center_axis',(-1.01338750660366E-31,1.26069923670246E-19,
1.));
#7344=DIRECTION('ref_axis',(1.,0.,0.));
#7345=DIRECTION('center_axis',(0.,0.,-1.));
#7346=DIRECTION('ref_axis',(1.,0.,0.));
#7347=DIRECTION('center_axis',(1.01338750660366E-31,-1.26069923670246E-19,
-1.));
#7348=DIRECTION('ref_axis',(1.,0.,0.));
#7349=DIRECTION('',(0.,0.,-1.));
#7350=DIRECTION('center_axis',(-1.01338750660366E-31,1.26069923670246E-19,
1.));
#7351=DIRECTION('ref_axis',(1.,0.,0.));
#7352=DIRECTION('center_axis',(0.,0.,-1.));
#7353=DIRECTION('ref_axis',(1.,0.,0.));
#7354=DIRECTION('center_axis',(1.01338750660366E-31,-1.26069923670246E-19,
-1.));
#7355=DIRECTION('ref_axis',(1.,0.,0.));
#7356=DIRECTION('',(0.,0.,-1.));
#7357=DIRECTION('center_axis',(-1.01338750660366E-31,1.26069923670246E-19,
1.));
#7358=DIRECTION('ref_axis',(1.,0.,0.));
#7359=DIRECTION('center_axis',(0.,0.,-1.));
#7360=DIRECTION('ref_axis',(1.,0.,0.));
#7361=DIRECTION('center_axis',(1.01338750660366E-31,-1.26069923670246E-19,
-1.));
#7362=DIRECTION('ref_axis',(1.,0.,0.));
#7363=DIRECTION('',(0.,0.,-1.));
#7364=DIRECTION('center_axis',(-1.01338750660366E-31,1.26069923670246E-19,
1.));
#7365=DIRECTION('ref_axis',(1.,0.,0.));
#7366=DIRECTION('center_axis',(0.,0.,-1.));
#7367=DIRECTION('ref_axis',(1.,0.,0.));
#7368=DIRECTION('center_axis',(1.01338750660366E-31,-1.26069923670246E-19,
-1.));
#7369=DIRECTION('ref_axis',(1.,0.,0.));
#7370=DIRECTION('',(0.,0.,-1.));
#7371=DIRECTION('center_axis',(0.,0.,-1.));
#7372=DIRECTION('ref_axis',(1.,0.,0.));
#7373=DIRECTION('center_axis',(0.,0.,-1.));
#7374=DIRECTION('ref_axis',(1.,0.,0.));
#7375=DIRECTION('center_axis',(0.,0.,1.));
#7376=DIRECTION('ref_axis',(1.,0.,0.));
#7377=DIRECTION('center_axis',(0.,0.,-1.));
#7378=DIRECTION('ref_axis',(1.,0.,0.));
#7379=DIRECTION('center_axis',(1.01338750660366E-31,-1.26069923670246E-19,
-1.));
#7380=DIRECTION('ref_axis',(1.,0.,0.));
#7381=DIRECTION('',(0.,0.,-1.));
#7382=DIRECTION('center_axis',(0.,0.,-1.));
#7383=DIRECTION('ref_axis',(1.,0.,0.));
#7384=DIRECTION('center_axis',(0.,0.,-1.));
#7385=DIRECTION('ref_axis',(1.,0.,0.));
#7386=DIRECTION('center_axis',(0.,0.,1.));
#7387=DIRECTION('ref_axis',(1.,0.,0.));
#7388=DIRECTION('center_axis',(0.,0.,-1.));
#7389=DIRECTION('ref_axis',(1.,0.,0.));
#7390=DIRECTION('',(0.,0.,-1.));
#7391=DIRECTION('center_axis',(0.,0.,1.));
#7392=DIRECTION('ref_axis',(1.,0.,0.));
#7393=DIRECTION('center_axis',(0.,0.,-1.));
#7394=DIRECTION('ref_axis',(1.,0.,0.));
#7395=DIRECTION('',(0.,0.,-1.));
#7396=DIRECTION('center_axis',(0.,0.,1.));
#7397=DIRECTION('ref_axis',(1.,0.,0.));
#7398=DIRECTION('center_axis',(0.,-1.,0.));
#7399=DIRECTION('ref_axis',(-1.,0.,0.));
#7400=DIRECTION('',(0.0523359562429438,0.,0.998629534754574));
#7401=DIRECTION('',(1.,0.,0.));
#7402=DIRECTION('',(-0.0523359562429438,0.,-0.998629534754574));
#7403=DIRECTION('',(1.,0.,0.));
#7404=DIRECTION('center_axis',(0.,-1.,0.));
#7405=DIRECTION('ref_axis',(-1.,0.,0.));
#7406=DIRECTION('',(0.,0.,-1.));
#7407=DIRECTION('',(1.,0.,0.));
#7408=DIRECTION('',(0.,0.,1.));
#7409=DIRECTION('',(1.,0.,0.));
#7410=DIRECTION('center_axis',(0.,-1.,0.));
#7411=DIRECTION('ref_axis',(-1.,0.,0.));
#7412=DIRECTION('',(0.,0.,-1.));
#7413=DIRECTION('',(1.,0.,0.));
#7414=DIRECTION('',(0.,0.,1.));
#7415=DIRECTION('',(1.,0.,0.));
#7416=DIRECTION('center_axis',(0.,-1.,0.));
#7417=DIRECTION('ref_axis',(-1.,0.,0.));
#7418=DIRECTION('',(0.,0.,-1.));
#7419=DIRECTION('',(1.,0.,0.));
#7420=DIRECTION('',(0.,0.,1.));
#7421=DIRECTION('',(1.,0.,0.));
#7422=DIRECTION('center_axis',(0.,1.,0.));
#7423=DIRECTION('ref_axis',(1.,0.,0.));
#7424=DIRECTION('',(-0.0523359562429438,0.,-0.998629534754574));
#7425=DIRECTION('',(-1.,0.,0.));
#7426=DIRECTION('',(0.0523359562429438,0.,0.998629534754574));
#7427=DIRECTION('',(-1.,0.,0.));
#7428=DIRECTION('center_axis',(0.,1.,0.));
#7429=DIRECTION('ref_axis',(1.,0.,0.));
#7430=DIRECTION('',(0.,0.,1.));
#7431=DIRECTION('',(-1.,0.,0.));
#7432=DIRECTION('',(0.,0.,-1.));
#7433=DIRECTION('',(-1.,0.,0.));
#7434=DIRECTION('center_axis',(0.,1.,0.));
#7435=DIRECTION('ref_axis',(1.,0.,0.));
#7436=DIRECTION('',(0.,0.,1.));
#7437=DIRECTION('',(-1.,0.,0.));
#7438=DIRECTION('',(0.,0.,-1.));
#7439=DIRECTION('',(-1.,0.,0.));
#7440=DIRECTION('center_axis',(0.,0.,1.));
#7441=DIRECTION('ref_axis',(1.,0.,0.));
#7442=DIRECTION('center_axis',(0.,0.,1.));
#7443=DIRECTION('ref_axis',(1.,0.,0.));
#7444=DIRECTION('center_axis',(0.,0.,1.));
#7445=DIRECTION('ref_axis',(1.,0.,0.));
#7446=DIRECTION('center_axis',(0.,0.,1.));
#7447=DIRECTION('ref_axis',(1.,0.,0.));
#7448=DIRECTION('center_axis',(0.,0.,1.));
#7449=DIRECTION('ref_axis',(1.,0.,0.));
#7450=DIRECTION('',(0.,1.,0.));
#7451=DIRECTION('',(0.,-1.,0.));
#7452=DIRECTION('center_axis',(0.,0.,1.));
#7453=DIRECTION('ref_axis',(1.,0.,0.));
#7454=DIRECTION('',(0.,-1.,0.));
#7455=DIRECTION('',(0.,1.,0.));
#7456=DIRECTION('center_axis',(0.,0.,1.));
#7457=DIRECTION('ref_axis',(1.,0.,0.));
#7458=DIRECTION('',(0.,-1.,0.));
#7459=DIRECTION('',(0.,1.,0.));
#7460=DIRECTION('center_axis',(0.,0.,1.));
#7461=DIRECTION('ref_axis',(1.,0.,0.));
#7462=DIRECTION('',(0.,-1.,0.));
#7463=DIRECTION('',(-1.,0.,0.));
#7464=DIRECTION('',(0.,1.,0.));
#7465=DIRECTION('center_axis',(0.,1.,0.));
#7466=DIRECTION('ref_axis',(1.,0.,0.));
#7467=DIRECTION('',(0.,0.,1.));
#7468=DIRECTION('',(-1.,0.,0.));
#7469=DIRECTION('',(0.,0.,-1.));
#7470=DIRECTION('center_axis',(-1.,0.,0.));
#7471=DIRECTION('ref_axis',(0.,-1.,0.));
#7472=DIRECTION('',(0.,-1.,0.));
#7473=DIRECTION('',(0.,-1.,1.26069923670246E-19));
#7474=DIRECTION('center_axis',(1.,0.,0.));
#7475=DIRECTION('ref_axis',(0.,1.,0.));
#7476=DIRECTION('',(0.,1.,0.));
#7477=DIRECTION('',(0.,1.,-1.26069923670246E-19));
#7478=DIRECTION('',(0.,1.,0.));
#7479=DIRECTION('center_axis',(1.,0.,0.));
#7480=DIRECTION('ref_axis',(0.,1.,0.));
#7481=DIRECTION('',(0.,1.,0.));
#7482=DIRECTION('',(0.,1.,-1.26069923670246E-19));
#7483=DIRECTION('',(0.,1.,0.));
#7484=DIRECTION('center_axis',(1.,0.,0.));
#7485=DIRECTION('ref_axis',(0.,1.,0.));
#7486=DIRECTION('',(0.,1.,0.));
#7487=DIRECTION('',(0.,1.,-1.26069923670246E-19));
#7488=DIRECTION('',(0.,1.,0.));
#7489=DIRECTION('center_axis',(0.998629534754574,0.,-0.0523359562429438));
#7490=DIRECTION('ref_axis',(-0.0523359562429438,0.,-0.998629534754574));
#7491=DIRECTION('',(0.,-1.,0.));
#7492=DIRECTION('',(6.6070447339401E-21,-1.,1.26069923670246E-19));
#7493=DIRECTION('',(0.,-1.,0.));
#7494=DIRECTION('center_axis',(0.,0.,1.));
#7495=DIRECTION('ref_axis',(1.,0.,0.));
#7496=DIRECTION('',(0.,-1.,0.));
#7497=DIRECTION('',(0.,-1.,0.));
#7498=DIRECTION('',(0.,-1.,0.));
#7499=DIRECTION('',(0.,1.,0.));
#7500=DIRECTION('',(0.,-1.,0.));
#7501=DIRECTION('',(0.,1.,0.));
#7502=DIRECTION('',(0.,-1.,0.));
#7503=DIRECTION('',(0.,-1.,0.));
#7504=DIRECTION('',(0.,-1.,0.));
#7505=DIRECTION('',(0.,1.,0.));
#7506=DIRECTION('',(0.,1.,0.));
#7507=DIRECTION('center_axis',(0.,0.,1.));
#7508=DIRECTION('ref_axis',(1.,0.,0.));
#7509=DIRECTION('center_axis',(-1.01338750660366E-31,1.26069923670246E-19,
1.));
#7510=DIRECTION('ref_axis',(1.,0.,0.));
#7511=DIRECTION('',(0.,0.,-1.));
#7512=DIRECTION('center_axis',(0.,0.,1.));
#7513=DIRECTION('ref_axis',(1.,0.,0.));
#7514=DIRECTION('center_axis',(-1.01338750660366E-31,1.26069923670246E-19,
1.));
#7515=DIRECTION('ref_axis',(1.,0.,0.));
#7516=DIRECTION('',(0.,0.,-1.));
#7517=DIRECTION('center_axis',(1.,0.,0.));
#7518=DIRECTION('ref_axis',(0.,1.,0.));
#7519=DIRECTION('',(0.,1.,-1.26069923670246E-19));
#7520=DIRECTION('center_axis',(0.995216631131787,0.0976926666577189,1.18580395612125E-14));
#7521=DIRECTION('ref_axis',(0.0975341006448478,-0.993601284365854,0.0569524970297685));
#7522=DIRECTION('center_axis',(-1.01338750660366E-31,1.26069923670246E-19,
1.));
#7523=DIRECTION('ref_axis',(1.,0.,1.01338750660366E-31));
#7524=DIRECTION('center_axis',(-1.01338750660366E-31,1.26069923670246E-19,
1.));
#7525=DIRECTION('ref_axis',(1.,0.,1.01338750660366E-31));
#7526=DIRECTION('',(-6.60704473394009E-21,-1.,1.26069923670246E-19));
#7527=DIRECTION('center_axis',(-1.,0.,0.));
#7528=DIRECTION('ref_axis',(0.,-1.,0.));
#7529=DIRECTION('',(0.,-1.,1.26069923670246E-19));
#7530=DIRECTION('center_axis',(-1.01338750660366E-31,1.26069923670246E-19,
1.));
#7531=DIRECTION('ref_axis',(1.,0.,1.01338750660366E-31));
#7532=DIRECTION('center_axis',(-1.,0.,0.));
#7533=DIRECTION('ref_axis',(0.,-1.,0.));
#7534=DIRECTION('',(0.,-1.,1.26069923670246E-19));
#7535=DIRECTION('center_axis',(-1.01338750660366E-31,1.26069923670246E-19,
1.));
#7536=DIRECTION('ref_axis',(1.,0.,1.01338750660366E-31));
#7537=DIRECTION('center_axis',(-1.,0.,0.));
#7538=DIRECTION('ref_axis',(0.,-1.,0.));
#7539=DIRECTION('',(0.,-1.,1.26069923670246E-19));
#7540=DIRECTION('center_axis',(-0.982258063247475,0.187534256031586,1.45403402392141E-15));
#7541=DIRECTION('ref_axis',(1.48029736616688E-15,0.,1.));
#7542=DIRECTION('center_axis',(-1.01338750660366E-31,1.26069923670246E-19,
1.));
#7543=DIRECTION('ref_axis',(1.,0.,1.01338750660366E-31));
#7544=DIRECTION('',(-6.6070447339401E-21,1.,-1.26069923670246E-19));
#7545=DIRECTION('center_axis',(-0.982258063247479,-0.187534256031562,9.14061384143289E-15));
#7546=DIRECTION('ref_axis',(-0.187187393251729,0.980441281772238,0.0607928680392112));
#7547=DIRECTION('center_axis',(-0.45173408531537,0.373496730537872,-0.810207694632559));
#7548=DIRECTION('ref_axis',(-0.624418441188311,0.516273298501642,0.586142893463867));
#7549=DIRECTION('center_axis',(-2.96465769266614E-15,1.,0.));
#7550=DIRECTION('ref_axis',(0.,0.,1.));
#7551=DIRECTION('center_axis',(0.0522655346583812,-0.0518587053130894,0.997285810873755));
#7552=DIRECTION('ref_axis',(-0.998629534754574,0.,0.0523359562429445));
#7553=DIRECTION('center_axis',(0.377681861983732,-0.843372107574977,0.38220400219391));
#7554=DIRECTION('ref_axis',(0.592794689304902,0.537329962094562,0.599892463836113));
#7555=DIRECTION('center_axis',(0.995216631131786,-0.0976926666577302,0.));
#7556=DIRECTION('ref_axis',(0.,0.,1.));
#7557=DIRECTION('center_axis',(-0.0522650609395843,-0.052032719242908,0.997276771780618));
#7558=DIRECTION('ref_axis',(0.0975341006448596,0.993601284365853,0.0569524970297681));
#7559=DIRECTION('center_axis',(1.55158195278682E-16,1.,-2.96059473233375E-15));
#7560=DIRECTION('ref_axis',(0.998629534754574,0.,0.0523359562429438));
#7561=DIRECTION('center_axis',(-0.45173408531537,-0.373496730537869,-0.810207694632561));
#7562=DIRECTION('ref_axis',(-0.624418441188315,-0.516273298501641,0.586142893463864));
#7563=DIRECTION('center_axis',(0.0522655346583823,0.0518587053130918,0.997285810873755));
#7564=DIRECTION('ref_axis',(-0.187187393251729,-0.980441281772238,0.0607928680392122));
#7565=DIRECTION('center_axis',(-2.71526841737693E-16,-1.,-5.18104078158406E-15));
#7566=DIRECTION('ref_axis',(-0.998629534754574,0.,0.0523359562429439));
#7567=DIRECTION('center_axis',(-6.6070447339401E-21,1.,-1.26069923670246E-19));
#7568=DIRECTION('ref_axis',(-0.688354575693753,0.,0.725374371012289));
#7569=DIRECTION('center_axis',(-0.377681861983722,-0.843372107574983,-0.382204002193908));
#7570=DIRECTION('ref_axis',(0.592794689304909,-0.537329962094554,0.599892463836112));
#7571=DIRECTION('center_axis',(-0.0522650609395818,0.0520327192429072,0.997276771780618));
#7572=DIRECTION('ref_axis',(0.998629534754574,0.,0.0523359562429431));
#7573=DIRECTION('center_axis',(2.96465769266612E-15,-1.,0.));
#7574=DIRECTION('ref_axis',(0.,0.,1.));
#7575=DIRECTION('center_axis',(-6.60704473394009E-21,-1.,1.26069923670246E-19));
#7576=DIRECTION('ref_axis',(0.688354575693758,0.,0.725374371012284));
#7577=DIRECTION('',(6.60704473394009E-21,1.,-1.26069923670246E-19));
#7578=DIRECTION('center_axis',(-0.998629534754574,0.,-0.0523359562429438));
#7579=DIRECTION('ref_axis',(-0.0523359562429438,0.,0.998629534754574));
#7580=DIRECTION('center_axis',(-0.45173408531537,0.373496730537872,-0.81020769463256));
#7581=DIRECTION('ref_axis',(-0.624418441188311,0.516273298501643,0.586142893463866));
#7582=DIRECTION('center_axis',(-2.96465769266614E-15,1.,0.));
#7583=DIRECTION('ref_axis',(0.,0.,1.));
#7584=DIRECTION('center_axis',(-0.982258063247479,-0.187534256031562,9.14061384143289E-15));
#7585=DIRECTION('ref_axis',(-0.187187393251729,0.980441281772238,0.0607928680392111));
#7586=DIRECTION('center_axis',(0.0522655346583812,-0.0518587053130894,0.997285810873755));
#7587=DIRECTION('ref_axis',(-0.998629534754574,0.,0.0523359562429445));
#7588=DIRECTION('center_axis',(0.377681861983731,-0.843372107574978,0.38220400219391));
#7589=DIRECTION('ref_axis',(0.592794689304906,0.537329962094559,0.599892463836111));
#7590=DIRECTION('center_axis',(0.995216631131786,-0.0976926666577302,0.));
#7591=DIRECTION('ref_axis',(0.,0.,1.));
#7592=DIRECTION('center_axis',(1.55158195278682E-16,1.,-2.96059473233375E-15));
#7593=DIRECTION('ref_axis',(0.998629534754574,0.,0.0523359562429438));
#7594=DIRECTION('center_axis',(-0.0522650609395843,-0.052032719242908,0.997276771780618));
#7595=DIRECTION('ref_axis',(0.0975341006448596,0.993601284365853,0.0569524970297681));
#7596=DIRECTION('center_axis',(-0.45173408531537,-0.373496730537868,-0.810207694632561));
#7597=DIRECTION('ref_axis',(-0.624418441188315,-0.516273298501641,0.586142893463864));
#7598=DIRECTION('center_axis',(-0.982258063247475,0.187534256031586,1.45403402392141E-15));
#7599=DIRECTION('ref_axis',(1.48029736616688E-15,0.,1.));
#7600=DIRECTION('center_axis',(-2.71526841737693E-16,-1.,-5.18104078158406E-15));
#7601=DIRECTION('ref_axis',(-0.998629534754574,0.,0.0523359562429439));
#7602=DIRECTION('center_axis',(0.0522655346583823,0.0518587053130918,0.997285810873755));
#7603=DIRECTION('ref_axis',(-0.187187393251729,-0.980441281772238,0.0607928680392122));
#7604=DIRECTION('center_axis',(-6.6070447339401E-21,1.,-1.26069923670246E-19));
#7605=DIRECTION('ref_axis',(-0.688354575693753,0.,0.725374371012289));
#7606=DIRECTION('',(6.6070447339401E-21,-1.,1.26069923670246E-19));
#7607=DIRECTION('',(-6.6070447339401E-21,1.,-1.26069923670246E-19));
#7608=DIRECTION('center_axis',(-0.377681861983727,-0.843372107574981,-0.382204002193907));
#7609=DIRECTION('ref_axis',(0.592794689304909,-0.537329962094554,0.599892463836112));
#7610=DIRECTION('center_axis',(-0.0522650609395818,0.0520327192429072,0.997276771780618));
#7611=DIRECTION('ref_axis',(0.998629534754574,0.,0.0523359562429431));
#7612=DIRECTION('center_axis',(2.96465769266612E-15,-1.,0.));
#7613=DIRECTION('ref_axis',(0.,0.,1.));
#7614=DIRECTION('center_axis',(0.995216631131787,0.0976926666577189,1.18580395612125E-14));
#7615=DIRECTION('ref_axis',(0.0975341006448478,-0.993601284365854,0.0569524970297685));
#7616=DIRECTION('center_axis',(-6.60704473394009E-21,-1.,1.26069923670246E-19));
#7617=DIRECTION('ref_axis',(0.688354575693758,0.,0.725374371012284));
#7618=DIRECTION('',(6.60704473394009E-21,1.,-1.26069923670246E-19));
#7619=DIRECTION('',(-6.60704473394009E-21,-1.,1.26069923670246E-19));
#7620=DIRECTION('center_axis',(0.998629534754574,0.,-0.0523359562429438));
#7621=DIRECTION('ref_axis',(-0.0523359562429438,0.,-0.998629534754574));
#7622=DIRECTION('center_axis',(-1.01338750660366E-31,1.26069923670246E-19,
1.));
#7623=DIRECTION('ref_axis',(1.,0.,1.01338750660366E-31));
#7624=DIRECTION('center_axis',(-0.998629534754574,0.,-0.0523359562429438));
#7625=DIRECTION('ref_axis',(-0.0523359562429438,0.,0.998629534754574));
#8696=CARTESIAN_POINT('',(0.,0.,0.));
#8697=CARTESIAN_POINT('Origin',(9.,-1.,0.8));
#8698=CARTESIAN_POINT('',(8.85,-1.,0.9));
#8699=CARTESIAN_POINT('Origin',(9.,-1.,0.9));
#8700=CARTESIAN_POINT('',(8.85,-1.,0.7));
#8701=CARTESIAN_POINT('',(8.85,-1.,0.8));
#8702=CARTESIAN_POINT('Origin',(9.,-1.,0.7));
#8703=CARTESIAN_POINT('Origin',(3.,-1.,0.8));
#8704=CARTESIAN_POINT('',(2.85,-1.,0.9));
#8705=CARTESIAN_POINT('Origin',(3.,-1.,0.9));
#8706=CARTESIAN_POINT('',(2.85,-1.,0.7));
#8707=CARTESIAN_POINT('',(2.85,-1.,0.8));
#8708=CARTESIAN_POINT('Origin',(3.,-1.,0.7));
#8709=CARTESIAN_POINT('Origin',(3.,1.,0.8));
#8710=CARTESIAN_POINT('',(2.85,1.,0.9));
#8711=CARTESIAN_POINT('Origin',(3.,1.,0.9));
#8712=CARTESIAN_POINT('',(2.85,1.,0.7));
#8713=CARTESIAN_POINT('',(2.85,1.,0.8));
#8714=CARTESIAN_POINT('Origin',(3.,1.,0.7));
#8715=CARTESIAN_POINT('Origin',(9.,1.,0.8));
#8716=CARTESIAN_POINT('',(8.85,1.,0.9));
#8717=CARTESIAN_POINT('Origin',(9.,1.,0.9));
#8718=CARTESIAN_POINT('',(8.85,1.,0.7));
#8719=CARTESIAN_POINT('',(8.85,1.,0.8));
#8720=CARTESIAN_POINT('Origin',(9.,1.,0.7));
#8721=CARTESIAN_POINT('Origin',(2.,0.,0.75));
#8722=CARTESIAN_POINT('',(1.7,3.67394039744206E-17,0.9));
#8723=CARTESIAN_POINT('Origin',(2.,0.,0.9));
#8724=CARTESIAN_POINT('',(1.7,3.67394039744206E-17,0.6));
#8725=CARTESIAN_POINT('',(1.7,3.67394039744206E-17,0.75));
#8726=CARTESIAN_POINT('Origin',(2.,0.,0.6));
#8727=CARTESIAN_POINT('Origin',(2.,0.,0.6));
#8728=CARTESIAN_POINT('',(1.83,-2.0818995585505E-17,0.6));
#8729=CARTESIAN_POINT('Origin',(2.,0.,0.6));
#8730=CARTESIAN_POINT('Origin',(10.,0.,0.75));
#8731=CARTESIAN_POINT('',(9.7,3.67394039744206E-17,0.9));
#8732=CARTESIAN_POINT('Origin',(10.,0.,0.9));
#8733=CARTESIAN_POINT('',(9.7,3.67394039744206E-17,0.6));
#8734=CARTESIAN_POINT('',(9.7,3.67394039744206E-17,0.75));
#8735=CARTESIAN_POINT('Origin',(10.,0.,0.6));
#8736=CARTESIAN_POINT('Origin',(10.,0.,0.6));
#8737=CARTESIAN_POINT('',(9.83,-2.0818995585505E-17,0.6));
#8738=CARTESIAN_POINT('Origin',(10.,0.,0.6));
#8739=CARTESIAN_POINT('Origin',(2.,0.,0.45));
#8740=CARTESIAN_POINT('',(1.83,-2.0818995585505E-17,0.32));
#8741=CARTESIAN_POINT('',(1.83,2.0818995585505E-17,0.45));
#8742=CARTESIAN_POINT('Origin',(2.,0.,0.32));
#8743=CARTESIAN_POINT('Origin',(10.,0.,0.45));
#8744=CARTESIAN_POINT('',(9.83,-2.0818995585505E-17,0.32));
#8745=CARTESIAN_POINT('',(9.83,2.0818995585505E-17,0.45));
#8746=CARTESIAN_POINT('Origin',(10.,0.,0.32));
#8747=CARTESIAN_POINT('Origin',(11.2,-0.62,0.32));
#8748=CARTESIAN_POINT('',(0.200274469199584,-0.62,0.));
#8749=CARTESIAN_POINT('',(0.217044958570157,-0.62,0.32));
#8750=CARTESIAN_POINT('',(0.223426876981161,-0.62,0.441774257530303));
#8751=CARTESIAN_POINT('',(0.,-0.62,0.));
#8752=CARTESIAN_POINT('',(8.63987299740311,-0.62,0.));
#8753=CARTESIAN_POINT('',(0.0167704893705732,-0.62,0.32));
#8754=CARTESIAN_POINT('',(0.0237009700302462,-0.62,0.452241448778892));
#8755=CARTESIAN_POINT('',(-0.1,-0.62,0.32));
#8756=CARTESIAN_POINT('Origin',(11.2,-0.62,0.32));
#8757=CARTESIAN_POINT('',(0.9,-0.62,0.32));
#8758=CARTESIAN_POINT('',(0.9,-0.62,0.));
#8759=CARTESIAN_POINT('',(0.9,-0.62,0.16));
#8760=CARTESIAN_POINT('',(1.1,-0.62,0.32));
#8761=CARTESIAN_POINT('',(-0.1,-0.62,0.32));
#8762=CARTESIAN_POINT('',(1.1,-0.62,0.));
#8763=CARTESIAN_POINT('',(1.1,-0.62,0.16));
#8764=CARTESIAN_POINT('',(8.63987299740311,-0.62,0.));
#8765=CARTESIAN_POINT('Origin',(11.2,-0.62,0.32));
#8766=CARTESIAN_POINT('',(3.9,-0.62,0.32));
#8767=CARTESIAN_POINT('',(3.9,-0.62,0.));
#8768=CARTESIAN_POINT('',(3.9,-0.62,0.16));
#8769=CARTESIAN_POINT('',(4.1,-0.62,0.32));
#8770=CARTESIAN_POINT('',(-0.1,-0.62,0.32));
#8771=CARTESIAN_POINT('',(4.1,-0.62,0.));
#8772=CARTESIAN_POINT('',(4.1,-0.62,0.16));
#8773=CARTESIAN_POINT('',(8.63987299740311,-0.62,0.));
#8774=CARTESIAN_POINT('Origin',(11.2,-0.62,0.32));
#8775=CARTESIAN_POINT('',(7.9,-0.62,0.32));
#8776=CARTESIAN_POINT('',(7.9,-0.62,0.));
#8777=CARTESIAN_POINT('',(7.9,-0.62,0.16));
#8778=CARTESIAN_POINT('',(8.1,-0.62,0.32));
#8779=CARTESIAN_POINT('',(-0.1,-0.62,0.32));
#8780=CARTESIAN_POINT('',(8.1,-0.62,0.));
#8781=CARTESIAN_POINT('',(8.1,-0.62,0.16));
#8782=CARTESIAN_POINT('',(8.63987299740311,-0.62,0.));
#8783=CARTESIAN_POINT('Origin',(-0.0999999999999996,0.62,0.32));
#8784=CARTESIAN_POINT('',(0.217044958570158,0.62,0.32));
#8785=CARTESIAN_POINT('',(0.200274469199586,0.62,0.));
#8786=CARTESIAN_POINT('',(0.207951231396534,0.62,0.146481348799182));
#8787=CARTESIAN_POINT('',(0.0167704893705736,0.62,0.32));
#8788=CARTESIAN_POINT('',(11.2,0.62,0.32));
#8789=CARTESIAN_POINT('',(0.,0.62,0.));
#8790=CARTESIAN_POINT('',(0.00822532444561912,0.62,0.156948540047771));
#8791=CARTESIAN_POINT('',(2.98987299740311,0.62,0.));
#8792=CARTESIAN_POINT('Origin',(-0.0999999999999996,0.62,0.32));
#8793=CARTESIAN_POINT('',(0.9,0.62,0.));
#8794=CARTESIAN_POINT('',(0.9,0.62,0.32));
#8795=CARTESIAN_POINT('',(0.9,0.62,0.16));
#8796=CARTESIAN_POINT('',(1.1,0.62,0.));
#8797=CARTESIAN_POINT('',(2.98987299740311,0.62,0.));
#8798=CARTESIAN_POINT('',(1.1,0.62,0.32));
#8799=CARTESIAN_POINT('',(1.1,0.62,0.16));
#8800=CARTESIAN_POINT('',(11.2,0.62,0.32));
#8801=CARTESIAN_POINT('Origin',(-0.0999999999999996,0.62,0.32));
#8802=CARTESIAN_POINT('',(3.9,0.62,0.));
#8803=CARTESIAN_POINT('',(3.9,0.62,0.32));
#8804=CARTESIAN_POINT('',(3.9,0.62,0.16));
#8805=CARTESIAN_POINT('',(4.1,0.62,0.));
#8806=CARTESIAN_POINT('',(2.98987299740311,0.62,0.));
#8807=CARTESIAN_POINT('',(4.1,0.62,0.32));
#8808=CARTESIAN_POINT('',(4.1,0.62,0.16));
#8809=CARTESIAN_POINT('',(11.2,0.62,0.32));
#8810=CARTESIAN_POINT('Origin',(5.55,0.,0.32));
#8811=CARTESIAN_POINT('',(1.6,-4.89858719658941E-17,0.32));
#8812=CARTESIAN_POINT('Origin',(2.,0.,0.32));
#8813=CARTESIAN_POINT('Origin',(5.55,0.,0.32));
#8814=CARTESIAN_POINT('',(9.6,-4.89858719658942E-17,0.32));
#8815=CARTESIAN_POINT('Origin',(10.,0.,0.32));
#8816=CARTESIAN_POINT('Origin',(5.55,0.,0.32));
#8817=CARTESIAN_POINT('',(0.217044958570157,-0.7,0.32));
#8818=CARTESIAN_POINT('',(0.0167704893705731,-0.7,0.32));
#8819=CARTESIAN_POINT('Origin',(5.55,0.,0.32));
#8820=CARTESIAN_POINT('',(0.9,0.724814814814815,0.32));
#8821=CARTESIAN_POINT('',(1.1,-0.724814814814815,0.32));
#8822=CARTESIAN_POINT('Origin',(5.55,0.,0.32));
#8823=CARTESIAN_POINT('',(3.9,0.883148148148148,0.32));
#8824=CARTESIAN_POINT('',(4.1,-0.883148148148148,0.32));
#8825=CARTESIAN_POINT('Origin',(5.55,0.,0.32));
#8826=CARTESIAN_POINT('',(7.9,0.62,0.32));
#8827=CARTESIAN_POINT('',(7.9,0.886851851851852,0.32));
#8828=CARTESIAN_POINT('',(8.1,0.62,0.32));
#8829=CARTESIAN_POINT('',(11.2,0.62,0.32));
#8830=CARTESIAN_POINT('',(8.1,-0.886851851851852,0.32));
#8831=CARTESIAN_POINT('Origin',(-0.0999999999999996,0.62,0.32));
#8832=CARTESIAN_POINT('',(7.9,0.62,0.));
#8833=CARTESIAN_POINT('',(7.9,0.62,0.16));
#8834=CARTESIAN_POINT('',(8.1,0.62,0.));
#8835=CARTESIAN_POINT('',(2.98987299740311,0.62,0.));
#8836=CARTESIAN_POINT('',(8.1,0.62,0.16));
#8837=CARTESIAN_POINT('Origin',(11.2,1.53779953703704,0.));
#8838=CARTESIAN_POINT('',(11.2,1.47592264243751,0.));
#8839=CARTESIAN_POINT('',(11.2,-1.47592264243751,0.));
#8840=CARTESIAN_POINT('',(11.2,1.53779953703704,0.));
#8841=CARTESIAN_POINT('',(11.2,-1.44160695250311,0.605635447211793));
#8842=CARTESIAN_POINT('Ctrl Pts',(11.2,-1.44160695250311,0.605635447211793));
#8843=CARTESIAN_POINT('Ctrl Pts',(11.2,-1.44733381480461,0.504614841520655));
#8844=CARTESIAN_POINT('Ctrl Pts',(11.2,-1.45305922122436,0.403593539811385));
#8845=CARTESIAN_POINT('Ctrl Pts',(11.2,-1.46449774781658,0.201715464978033));
#8846=CARTESIAN_POINT('Ctrl Pts',(11.2,-1.47021094199039,0.100857470386242));
#8847=CARTESIAN_POINT('Ctrl Pts',(11.2,-1.47592264243751,0.));
#8848=CARTESIAN_POINT('',(11.2,-1.3413305091784,0.7));
#8849=CARTESIAN_POINT('Ctrl Pts',(11.2,-1.34133050917871,0.7));
#8850=CARTESIAN_POINT('Ctrl Pts',(11.2,-1.34927184579059,0.7));
#8851=CARTESIAN_POINT('Ctrl Pts',(11.1999981201149,-1.35715077597425,0.699006225306896));
#8852=CARTESIAN_POINT('Ctrl Pts',(11.1999964866412,-1.36482619101963,0.697118463987577));
#8853=CARTESIAN_POINT('Ctrl Pts',(11.1999955714568,-1.36912648693643,0.696060810134936));
#8854=CARTESIAN_POINT('Ctrl Pts',(11.1999947385598,-1.37336294684024,0.694721504600825));
#8855=CARTESIAN_POINT('Ctrl Pts',(11.1999942054834,-1.37750904339755,0.693111246644731));
#8856=CARTESIAN_POINT('Ctrl Pts',(11.1999932489192,-1.38494889279378,0.690221763364053));
#8857=CARTESIAN_POINT('Ctrl Pts',(11.1999934335488,-1.39201911070639,0.686493604183975));
#8858=CARTESIAN_POINT('Ctrl Pts',(11.1999946360439,-1.39857284316731,0.682006025455124));
#8859=CARTESIAN_POINT('Ctrl Pts',(11.1999952980149,-1.40218065925828,0.679535622697003));
#8860=CARTESIAN_POINT('Ctrl Pts',(11.1999962427007,-1.40563167682227,0.676834205328214));
#8861=CARTESIAN_POINT('Ctrl Pts',(11.1999970766466,-1.40889738828709,0.673909521834337));
#8862=CARTESIAN_POINT('Ctrl Pts',(11.1999978839828,-1.41205889660265,0.671078159882768));
#8863=CARTESIAN_POINT('Ctrl Pts',(11.1999985961359,-1.41502771690814,0.668054510912379));
#8864=CARTESIAN_POINT('Ctrl Pts',(11.1999985943254,-1.41778154893794,0.664849526385156));
#8865=CARTESIAN_POINT('Ctrl Pts',(11.1999985909468,-1.42292039881534,0.658868793295219));
#8866=CARTESIAN_POINT('Ctrl Pts',(11.1999963776609,-1.42731355725865,0.652257958652517));
#8867=CARTESIAN_POINT('Ctrl Pts',(11.1999956369,-1.43089859237711,0.645180832176479));
#8868=CARTESIAN_POINT('Ctrl Pts',(11.1999955610412,-1.43126572346771,0.644456088045497));
#8869=CARTESIAN_POINT('Ctrl Pts',(11.1999954968237,-1.43162433912915,0.643726434786758));
#8870=CARTESIAN_POINT('Ctrl Pts',(11.1999954455063,-1.43197434355081,0.642992037678167));
#8871=CARTESIAN_POINT('Ctrl Pts',(11.1999949451572,-1.43538691836834,0.635831599341589));
#8872=CARTESIAN_POINT('Ctrl Pts',(11.1999960935741,-1.43794480573841,0.628305806294037));
#8873=CARTESIAN_POINT('Ctrl Pts',(11.1999977538348,-1.43959303921538,0.620581877990282));
#8874=CARTESIAN_POINT('Ctrl Pts',(11.1999988103007,-1.44064185190664,0.615666946856702));
#8875=CARTESIAN_POINT('Ctrl Pts',(11.1999999935832,-1.44132148083109,0.610671141596651));
#8876=CARTESIAN_POINT('Ctrl Pts',(11.1999999950647,-1.44160695392865,0.605635447210179));
#8877=CARTESIAN_POINT('',(11.2,1.34133050917871,0.7));
#8878=CARTESIAN_POINT('',(11.2,0.768899768518519,0.7));
#8879=CARTESIAN_POINT('',(11.2,1.44160695250311,0.605635447211793));
#8880=CARTESIAN_POINT('Ctrl Pts',(11.1999999950647,1.44160695392865,0.605635447210179));
#8881=CARTESIAN_POINT('Ctrl Pts',(11.1999999927383,1.44115867123275,0.613543073794128));
#8882=CARTESIAN_POINT('Ctrl Pts',(11.199997327584,1.43974095598264,0.62135504174347));
#8883=CARTESIAN_POINT('Ctrl Pts',(11.1999961426836,1.43743894790867,0.628911795513178));
#8884=CARTESIAN_POINT('Ctrl Pts',(11.1999954950047,1.43618064644969,0.633042395401645));
#8885=CARTESIAN_POINT('Ctrl Pts',(11.1999951984378,1.4346571631488,0.63709676955888));
#8886=CARTESIAN_POINT('Ctrl Pts',(11.1999953420225,1.43287614971348,0.641047046155727));
#8887=CARTESIAN_POINT('Ctrl Pts',(11.1999956050472,1.42961361303411,0.648283331988978));
#8888=CARTESIAN_POINT('Ctrl Pts',(11.1999975633633,1.42552584716917,0.655091209244077));
#8889=CARTESIAN_POINT('Ctrl Pts',(11.1999983488166,1.42067941835906,0.661308913390503));
#8890=CARTESIAN_POINT('Ctrl Pts',(11.1999985007599,1.41974189284539,0.662511707551344));
#8891=CARTESIAN_POINT('Ctrl Pts',(11.1999985958742,1.41877583892185,0.663692344451305));
#8892=CARTESIAN_POINT('Ctrl Pts',(11.1999985956185,1.41778154881703,0.664849526385225));
#8893=CARTESIAN_POINT('Ctrl Pts',(11.199998595152,1.41596832836708,0.666959801783445));
#8894=CARTESIAN_POINT('Ctrl Pts',(11.1999982799021,1.41406123008998,0.668992111776222));
#8895=CARTESIAN_POINT('Ctrl Pts',(11.1999978412043,1.41206657472189,0.670943322037058));
#8896=CARTESIAN_POINT('Ctrl Pts',(11.1999965906985,1.40638082038708,0.676505236328724));
#8897=CARTESIAN_POINT('Ctrl Pts',(11.1999945592311,1.40005057587654,0.681348449922958));
#8898=CARTESIAN_POINT('Ctrl Pts',(11.1999938793032,1.39324090595796,0.685420973467861));
#8899=CARTESIAN_POINT('Ctrl Pts',(11.1999934424014,1.38886521116801,0.68803785802621));
#8900=CARTESIAN_POINT('Ctrl Pts',(11.1999934711477,1.38429057260668,0.690335857752236));
#8901=CARTESIAN_POINT('Ctrl Pts',(11.1999939665515,1.37955471147715,0.692291686537622));
#8902=CARTESIAN_POINT('Ctrl Pts',(11.1999947349645,1.37220899016913,0.695325342464331));
#8903=CARTESIAN_POINT('Ctrl Pts',(11.1999966395725,1.36455954597093,0.697503651902993));
#8904=CARTESIAN_POINT('Ctrl Pts',(11.1999981885915,1.35675452105021,0.698758058199902));
#8905=CARTESIAN_POINT('Ctrl Pts',(11.1999991983045,1.35166689148409,0.699575730741489));
#8906=CARTESIAN_POINT('Ctrl Pts',(11.2,1.34651254223162,0.7));
#8907=CARTESIAN_POINT('Ctrl Pts',(11.2,1.34133050917871,0.7));
#8908=CARTESIAN_POINT('Ctrl Pts',(11.2,1.47592264243751,0.));
#8909=CARTESIAN_POINT('Ctrl Pts',(11.2,1.47021025951677,0.100869521536925));
#8910=CARTESIAN_POINT('Ctrl Pts',(11.2,1.4644963825062,0.20173956751342));
#8911=CARTESIAN_POINT('Ctrl Pts',(11.2,1.45305785520703,0.403617642353031));
#8912=CARTESIAN_POINT('Ctrl Pts',(11.2,1.44733313162379,0.50462689268162));
#8913=CARTESIAN_POINT('Ctrl Pts',(11.2,1.44160695250311,0.605635447211793));
#8914=CARTESIAN_POINT('Origin',(8.1,-1.7737037037037,0.));
#8915=CARTESIAN_POINT('',(8.1,1.69866351109718,0.));
#8916=CARTESIAN_POINT('',(8.1,-1.7737037037037,0.));
#8917=CARTESIAN_POINT('',(8.1,1.66641703131627,0.605314487869832));
#8918=CARTESIAN_POINT('Ctrl Pts',(8.1,1.66641703131627,0.605314487869832));
#8919=CARTESIAN_POINT('Ctrl Pts',(8.1,1.67178339996556,0.504592280948055));
#8920=CARTESIAN_POINT('Ctrl Pts',(8.1,1.67714947719849,0.403869246528492));
#8921=CARTESIAN_POINT('Ctrl Pts',(8.1,1.68789827452893,0.202098297941347));
#8922=CARTESIAN_POINT('Ctrl Pts',(8.1,1.69328107955938,0.101048748975501));
#8923=CARTESIAN_POINT('Ctrl Pts',(8.1,1.69866351109718,0.));
#8924=CARTESIAN_POINT('',(8.1,1.56644778183753,0.7));
#8925=CARTESIAN_POINT('Ctrl Pts',(8.0999999986552,1.56644778212326,0.7));
#8926=CARTESIAN_POINT('Ctrl Pts',(8.10000000155239,1.57436337254628,0.699999999341293));
#8927=CARTESIAN_POINT('Ctrl Pts',(8.09999905041684,1.58221543358893,0.699005989267703));
#8928=CARTESIAN_POINT('Ctrl Pts',(8.09999821745812,1.58986365929578,0.697118696434997));
#8929=CARTESIAN_POINT('Ctrl Pts',(8.099997748439,1.59417019217574,0.69605600700222));
#8930=CARTESIAN_POINT('Ctrl Pts',(8.09999731997616,1.59841215407948,0.694709061504878));
#8931=CARTESIAN_POINT('Ctrl Pts',(8.09999704681388,1.60256279759721,0.693088866918468));
#8932=CARTESIAN_POINT('Ctrl Pts',(8.09999655811104,1.60998853482381,0.690190246691698));
#8933=CARTESIAN_POINT('Ctrl Pts',(8.09999665589197,1.61704187682962,0.686451534538094));
#8934=CARTESIAN_POINT('Ctrl Pts',(8.09999726576867,1.62357667434142,0.681954089017224));
#8935=CARTESIAN_POINT('Ctrl Pts',(8.09999760196939,1.62717904774802,0.679474826559159));
#8936=CARTESIAN_POINT('Ctrl Pts',(8.09999808150314,1.6306235748906,0.676764109620253));
#8937=CARTESIAN_POINT('Ctrl Pts',(8.09999850764167,1.63388182210815,0.673830012183301));
#8938=CARTESIAN_POINT('Ctrl Pts',(8.09999892160867,1.637047006066,0.670979719520364));
#8939=CARTESIAN_POINT('Ctrl Pts',(8.09999928906958,1.640017230617,0.667935813742119));
#8940=CARTESIAN_POINT('Ctrl Pts',(8.09999928944056,1.64277007752663,0.664709670235875));
#8941=CARTESIAN_POINT('Ctrl Pts',(8.09999929012967,1.64788359851353,0.658716982277737));
#8942=CARTESIAN_POINT('Ctrl Pts',(8.09999816327153,1.65225000627493,0.652096887528603));
#8943=CARTESIAN_POINT('Ctrl Pts',(8.09999778355904,1.65580927004486,0.645014643130784));
#8944=CARTESIAN_POINT('Ctrl Pts',(8.09999774450894,1.65617530914943,0.644286296325024));
#8945=CARTESIAN_POINT('Ctrl Pts',(8.09999771143612,1.65653277094855,0.643553041785202));
#8946=CARTESIAN_POINT('Ctrl Pts',(8.0999976850083,1.65688156115921,0.642815048027137));
#8947=CARTESIAN_POINT('Ctrl Pts',(8.09999742811004,1.66027206465027,0.635641192980042));
#8948=CARTESIAN_POINT('Ctrl Pts',(8.09999800724182,1.66280786743682,0.628104262855387));
#8949=CARTESIAN_POINT('Ctrl Pts',(8.09999885110511,1.66443535430957,0.620372450280339));
#8950=CARTESIAN_POINT('Ctrl Pts',(8.09999939164969,1.6654778563549,0.615419764910946));
#8951=CARTESIAN_POINT('Ctrl Pts',(8.1,1.66614680274328,0.610386449940169));
#8952=CARTESIAN_POINT('Ctrl Pts',(8.1,1.66641703131627,0.605314487869832));
#8953=CARTESIAN_POINT('',(8.1,-1.56644778183827,0.7));
#8954=CARTESIAN_POINT('',(8.1,-0.886851851851852,0.7));
#8955=CARTESIAN_POINT('',(8.1,-1.66641703131627,0.605314487869832));
#8956=CARTESIAN_POINT('Ctrl Pts',(8.1,-1.66641703131627,0.605314487869832));
#8957=CARTESIAN_POINT('Ctrl Pts',(8.1,-1.66599546653325,0.613226902778437));
#8958=CARTESIAN_POINT('Ctrl Pts',(8.09999864563672,-1.66460605882141,0.621047760783158));
#8959=CARTESIAN_POINT('Ctrl Pts',(8.09999804140045,-1.66233302739118,0.628616817026045));
#8960=CARTESIAN_POINT('Ctrl Pts',(8.09999770486592,-1.66106704316887,0.632832467392296));
#8961=CARTESIAN_POINT('Ctrl Pts',(8.0999975536836,-1.65952595995304,0.636970042829054));
#8962=CARTESIAN_POINT('Ctrl Pts',(8.09999763427866,-1.65771765414013,0.640999885518982));
#8963=CARTESIAN_POINT('Ctrl Pts',(8.09999777898787,-1.65447082344915,0.64823550729937));
#8964=CARTESIAN_POINT('Ctrl Pts',(8.09999878245444,-1.65040085231772,0.655045563401426));
#8965=CARTESIAN_POINT('Ctrl Pts',(8.09999917121848,-1.64557198994432,0.661267087195486));
#8966=CARTESIAN_POINT('Ctrl Pts',(8.09999924425118,-1.6446648462537,0.662435854416292));
#8967=CARTESIAN_POINT('Ctrl Pts',(8.09999928944999,-1.64373079085321,0.663583781603691));
#8968=CARTESIAN_POINT('Ctrl Pts',(8.09999928890117,-1.64277007755202,0.664709670235858));
#8969=CARTESIAN_POINT('Ctrl Pts',(8.09999928782175,-1.64088054556816,0.666924069243459));
#8970=CARTESIAN_POINT('Ctrl Pts',(8.09999911129818,-1.63888792496677,0.66905326411728));
#8971=CARTESIAN_POINT('Ctrl Pts',(8.09999887085824,-1.63679941630975,0.671093569621172));
#8972=CARTESIAN_POINT('Ctrl Pts',(8.09999821641022,-1.6311147520694,0.676647030794692));
#8973=CARTESIAN_POINT('Ctrl Pts',(8.0999972000003,-1.62478663867955,0.681482189379454));
#8974=CARTESIAN_POINT('Ctrl Pts',(8.09999686812141,-1.6179789612855,0.685544965666037));
#8975=CARTESIAN_POINT('Ctrl Pts',(8.09999665686968,-1.61364565292072,0.68813105508359));
#8976=CARTESIAN_POINT('Ctrl Pts',(8.09999667786582,-1.6091170759025,0.690403516124292));
#8977=CARTESIAN_POINT('Ctrl Pts',(8.0999969341683,-1.60442977212996,0.692339085768374));
#8978=CARTESIAN_POINT('Ctrl Pts',(8.09999733452329,-1.59710801128849,0.695362524980696));
#8979=CARTESIAN_POINT('Ctrl Pts',(8.09999831212369,-1.58948382509795,0.697531565976904));
#8980=CARTESIAN_POINT('Ctrl Pts',(8.09999909563861,-1.58170429192971,0.698776637084609));
#8981=CARTESIAN_POINT('Ctrl Pts',(8.09999960249138,-1.57667174192468,0.69958206878261));
#8982=CARTESIAN_POINT('Ctrl Pts',(8.1000000005313,-1.5715735875011,0.699999999573449));
#8983=CARTESIAN_POINT('Ctrl Pts',(8.0999999986552,-1.56644778212326,0.7));
#8984=CARTESIAN_POINT('',(8.1,-1.69866351109718,0.));
#8985=CARTESIAN_POINT('Ctrl Pts',(8.1,-1.69866351109718,0.));
#8986=CARTESIAN_POINT('Ctrl Pts',(8.1,-1.69328105674055,0.101049177371948));
#8987=CARTESIAN_POINT('Ctrl Pts',(8.1,-1.68789822886868,0.202099155105557));
#8988=CARTESIAN_POINT('Ctrl Pts',(8.1,-1.67714943151225,0.403870104074094));
#8989=CARTESIAN_POINT('Ctrl Pts',(8.1,-1.67178337712185,0.50459270970527));
#8990=CARTESIAN_POINT('Ctrl Pts',(8.1,-1.66641703131627,0.605314487869832));
#8991=CARTESIAN_POINT('',(8.1,-1.7737037037037,0.));
#8992=CARTESIAN_POINT('Origin',(4.1,-1.7662962962963,0.));
#8993=CARTESIAN_POINT('',(4.1,1.70113889814581,0.));
#8994=CARTESIAN_POINT('',(4.1,-1.7662962962963,0.));
#8995=CARTESIAN_POINT('',(4.1,1.66887738702937,0.605315322680072));
#8996=CARTESIAN_POINT('Ctrl Pts',(4.1,1.66887738702937,0.605315322680072));
#8997=CARTESIAN_POINT('Ctrl Pts',(4.1,1.67424235111642,0.50466767694528));
#8998=CARTESIAN_POINT('Ctrl Pts',(4.1,1.67960699363804,0.404019058341251));
#8999=CARTESIAN_POINT('Ctrl Pts',(4.1,1.69036079691899,0.202247931921761));
#9000=CARTESIAN_POINT('Ctrl Pts',(4.1,1.6957500571643,0.101123491803998));
#9001=CARTESIAN_POINT('Ctrl Pts',(4.1,1.70113889814581,0.));
#9002=CARTESIAN_POINT('',(4.1,1.56887583540973,0.7));
#9003=CARTESIAN_POINT('Ctrl Pts',(4.1,1.56887583540973,0.7));
#9004=CARTESIAN_POINT('Ctrl Pts',(4.1,1.57679416129392,0.7));
#9005=CARTESIAN_POINT('Ctrl Pts',(4.10000107724674,1.58464912207822,0.699006028000541));
#9006=CARTESIAN_POINT('Ctrl Pts',(4.10000201939527,1.59230028572239,0.697118705459362));
#9007=CARTESIAN_POINT('Ctrl Pts',(4.10000255022779,1.59661116283941,0.696055335763773));
#9008=CARTESIAN_POINT('Ctrl Pts',(4.10000303435977,1.60085740028891,0.694707333985525));
#9009=CARTESIAN_POINT('Ctrl Pts',(4.10000334030352,1.60501217339351,0.693085708041268));
#9010=CARTESIAN_POINT('Ctrl Pts',(4.10000388718746,1.61243895913315,0.690187001388783));
#9011=CARTESIAN_POINT('Ctrl Pts',(4.10000376557609,1.61949349263125,0.686448444730844));
#9012=CARTESIAN_POINT('Ctrl Pts',(4.10000306534783,1.6260295229635,0.681951159450519));
#9013=CARTESIAN_POINT('Ctrl Pts',(4.10000267892397,1.62963645835533,0.679469313954069));
#9014=CARTESIAN_POINT('Ctrl Pts',(4.10000213012555,1.63308521926452,0.676755517937216));
#9015=CARTESIAN_POINT('Ctrl Pts',(4.1000016436875,1.63634725251217,0.673817835781739));
#9016=CARTESIAN_POINT('Ctrl Pts',(4.10000117237165,1.63950787692018,0.67097147916344));
#9017=CARTESIAN_POINT('Ctrl Pts',(4.10000075597222,1.64247408874941,0.667932078875657));
#9018=CARTESIAN_POINT('Ctrl Pts',(4.10000075698646,1.64522354659423,0.664710927554201));
#9019=CARTESIAN_POINT('Ctrl Pts',(4.1000007588733,1.65033845220459,0.658718515269377));
#9020=CARTESIAN_POINT('Ctrl Pts',(4.10000204656096,1.65470614797426,0.652098486008568));
#9021=CARTESIAN_POINT('Ctrl Pts',(4.10000248678323,1.65826650381873,0.645016049251367));
#9022=CARTESIAN_POINT('Ctrl Pts',(4.10000253228732,1.65863452415637,0.644283964909082));
#9023=CARTESIAN_POINT('Ctrl Pts',(4.10000257095464,1.65899387729575,0.643546919913709));
#9024=CARTESIAN_POINT('Ctrl Pts',(4.10000260201855,1.65934446736461,0.642805085364403));
#9025=CARTESIAN_POINT('Ctrl Pts',(4.10000290242009,1.66273482600052,0.635631222228741));
#9026=CARTESIAN_POINT('Ctrl Pts',(4.10000225562543,1.66527033938482,0.628094305374488));
#9027=CARTESIAN_POINT('Ctrl Pts',(4.10000130084992,1.66689736875237,0.62036252267401));
#9028=CARTESIAN_POINT('Ctrl Pts',(4.10000068968835,1.66793884687677,0.615413329558163));
#9029=CARTESIAN_POINT('Ctrl Pts',(4.09999999901039,1.66860722297681,0.610383627857512));
#9030=CARTESIAN_POINT('Ctrl Pts',(4.09999999630223,1.66887738567036,0.60531532268817));
#9031=CARTESIAN_POINT('',(4.1,-1.56887583540947,0.7));
#9032=CARTESIAN_POINT('',(4.1,-0.883148148148148,0.7));
#9033=CARTESIAN_POINT('',(4.1,-1.66887738702937,0.605315322680072));
#9034=CARTESIAN_POINT('Ctrl Pts',(4.09999999630223,-1.66887738567036,0.60531532268817));
#9035=CARTESIAN_POINT('Ctrl Pts',(4.10000000053001,-1.66845562780346,0.613227583070809));
#9036=CARTESIAN_POINT('Ctrl Pts',(4.10000153668442,-1.66706589531621,0.621048261667561));
#9037=CARTESIAN_POINT('Ctrl Pts',(4.10000221487211,-1.66479240287642,0.628617079688242));
#9038=CARTESIAN_POINT('Ctrl Pts',(4.10000259231836,-1.6635270876889,0.632829515245766));
#9039=CARTESIAN_POINT('Ctrl Pts',(4.10000275805793,-1.66198703315979,0.636963972243471));
#9040=CARTESIAN_POINT('Ctrl Pts',(4.10000266178038,-1.66018010017296,0.640990858692597));
#9041=CARTESIAN_POINT('Ctrl Pts',(4.10000248876893,-1.65693302887506,0.648227201990446));
#9042=CARTESIAN_POINT('Ctrl Pts',(4.10000134097948,-1.65286254930452,0.655037795911226));
#9043=CARTESIAN_POINT('Ctrl Pts',(4.100000893742,-1.6480330317196,0.661259713776781));
#9044=CARTESIAN_POINT('Ctrl Pts',(4.10000080951506,-1.647123502594,0.662431469633614));
#9045=CARTESIAN_POINT('Ctrl Pts',(4.10000075717637,-1.6461869221106,0.663582276554164));
#9046=CARTESIAN_POINT('Ctrl Pts',(4.10000075728519,-1.64522354661022,0.66471092755419));
#9047=CARTESIAN_POINT('Ctrl Pts',(4.10000075749815,-1.64333815989002,0.666919768869269));
#9048=CARTESIAN_POINT('Ctrl Pts',(4.1000009568795,-1.64135017761634,0.669043797975229));
#9049=CARTESIAN_POINT('Ctrl Pts',(4.10000122972053,-1.63926675509047,0.671079366787198));
#9050=CARTESIAN_POINT('Ctrl Pts',(4.10000197419082,-1.6335819569127,0.676633591976433));
#9051=CARTESIAN_POINT('Ctrl Pts',(4.10000313643093,-1.62725355063421,0.681469444454218));
#9052=CARTESIAN_POINT('Ctrl Pts',(4.1000035230587,-1.62044557755217,0.685533082105531));
#9053=CARTESIAN_POINT('Ctrl Pts',(4.10000376939409,-1.61610795658125,0.688122181633714));
#9054=CARTESIAN_POINT('Ctrl Pts',(4.10000375220654,-1.61157469281532,0.690397125746379));
#9055=CARTESIAN_POINT('Ctrl Pts',(4.10000346632868,-1.60688245467732,0.692334655286926));
#9056=CARTESIAN_POINT('Ctrl Pts',(4.10000302008581,-1.59955807566073,0.695359054367588));
#9057=CARTESIAN_POINT('Ctrl Pts',(4.1000019139068,-1.59193114173487,0.69752894708864));
#9058=CARTESIAN_POINT('Ctrl Pts',(4.10000102635309,-1.58414888227482,0.698774888159427));
#9059=CARTESIAN_POINT('Ctrl Pts',(4.10000045177616,-1.57911086966871,0.699581474839467));
#9060=CARTESIAN_POINT('Ctrl Pts',(4.1,-1.57400716417114,0.7));
#9061=CARTESIAN_POINT('Ctrl Pts',(4.1,-1.56887583540973,0.7));
#9062=CARTESIAN_POINT('',(4.1,-1.70113889814582,0.));
#9063=CARTESIAN_POINT('Ctrl Pts',(4.1,-1.70113889814582,0.));
#9064=CARTESIAN_POINT('Ctrl Pts',(4.1,-1.69575004793467,0.101123665001254));
#9065=CARTESIAN_POINT('Ctrl Pts',(4.1,-1.69036077845691,0.202248278345555));
#9066=CARTESIAN_POINT('Ctrl Pts',(4.1,-1.67960697517202,0.404019404791024));
#9067=CARTESIAN_POINT('Ctrl Pts',(4.1,-1.67424234188296,0.504667850166609));
#9068=CARTESIAN_POINT('Ctrl Pts',(4.1,-1.66887738702937,0.605315322680072));
#9069=CARTESIAN_POINT('',(4.1,-1.7662962962963,0.));
#9070=CARTESIAN_POINT('Origin',(1.1,-1.44962962962963,0.));
#9071=CARTESIAN_POINT('',(1.1,1.39262953588351,0.));
#9072=CARTESIAN_POINT('',(1.1,-1.44962962962963,0.));
#9073=CARTESIAN_POINT('',(1.10000000000005,1.35674377243284,0.605845626926786));
#9074=CARTESIAN_POINT('Ctrl Pts',(1.10000000000005,1.35674377243284,0.605845626926786));
#9075=CARTESIAN_POINT('Ctrl Pts',(1.10000000000005,1.36273568520883,0.504787121979256));
#9076=CARTESIAN_POINT('Ctrl Pts',(1.1,1.36872466312622,0.403727404115485));
#9077=CARTESIAN_POINT('Ctrl Pts',(1.1,1.38068651056748,0.201779555185378));
#9078=CARTESIAN_POINT('Ctrl Pts',(1.1,1.38665951284069,0.10088935150083));
#9079=CARTESIAN_POINT('Ctrl Pts',(1.1,1.39262953588351,0.));
#9080=CARTESIAN_POINT('',(1.1,1.25565664448622,0.7));
#9081=CARTESIAN_POINT('Ctrl Pts',(1.1,1.25565664448621,0.7));
#9082=CARTESIAN_POINT('Ctrl Pts',(1.1,1.26365753466764,0.700000000000001));
#9083=CARTESIAN_POINT('Ctrl Pts',(1.10000312127109,1.27160078819195,0.699008097631352));
#9084=CARTESIAN_POINT('Ctrl Pts',(1.10000579554281,1.27934333527045,0.697120485426804));
#9085=CARTESIAN_POINT('Ctrl Pts',(1.10000709386889,1.28310224676699,0.696204072889075));
#9086=CARTESIAN_POINT('Ctrl Pts',(1.10000828779753,1.28681383019745,0.695075712339665));
#9087=CARTESIAN_POINT('Ctrl Pts',(1.10000913303706,1.29046059826345,0.693742188764313));
#9088=CARTESIAN_POINT('Ctrl Pts',(1.10001087659788,1.29798315455626,0.69099139518989));
#9089=CARTESIAN_POINT('Ctrl Pts',(1.10001086910546,1.30515375246939,0.687398976275641));
#9090=CARTESIAN_POINT('Ctrl Pts',(1.10000899624477,1.31182501206943,0.683041610144935));
#9091=CARTESIAN_POINT('Ctrl Pts',(1.10000779407289,1.31610723164143,0.680244657298552));
#9092=CARTESIAN_POINT('Ctrl Pts',(1.10000585478529,1.32018349952736,0.677131483611404));
#9093=CARTESIAN_POINT('Ctrl Pts',(1.10000422180804,1.32400796947387,0.673713330684339));
#9094=CARTESIAN_POINT('Ctrl Pts',(1.10000291018178,1.3270798280974,0.670967830603965));
#9095=CARTESIAN_POINT('Ctrl Pts',(1.10000180047651,1.32997084712789,0.668041731908725));
#9096=CARTESIAN_POINT('Ctrl Pts',(1.10000182449184,1.33266034096938,0.664944387470286));
#9097=CARTESIAN_POINT('Ctrl Pts',(1.10000187074845,1.33784065079383,0.65897850512594));
#9098=CARTESIAN_POINT('Ctrl Pts',(1.10000564109429,1.34227630326151,0.652378581761819));
#9099=CARTESIAN_POINT('Ctrl Pts',(1.10000696187003,1.34590032739451,0.645305437365917));
#9100=CARTESIAN_POINT('Ctrl Pts',(1.100007110355,1.34630774940504,0.644510256482779));
#9101=CARTESIAN_POINT('Ctrl Pts',(1.10000723579819,1.34670486410349,0.643709073603569));
#9102=CARTESIAN_POINT('Ctrl Pts',(1.10000733566964,1.34709153749004,0.642902104572485));
#9103=CARTESIAN_POINT('Ctrl Pts',(1.10000822022419,1.35051627708745,0.63575483535061));
#9104=CARTESIAN_POINT('Ctrl Pts',(1.10000635568239,1.35308446649167,0.628241602461225));
#9105=CARTESIAN_POINT('Ctrl Pts',(1.10000361780323,1.35473867947858,0.620527690691125));
#9106=CARTESIAN_POINT('Ctrl Pts',(1.1000019043033,1.35577396762308,0.615699943921843));
#9107=CARTESIAN_POINT('Ctrl Pts',(1.09999998677418,1.35645041192828,0.610792997969602));
#9108=CARTESIAN_POINT('Ctrl Pts',(1.09999997754868,1.35674374570294,0.605845627052288));
#9109=CARTESIAN_POINT('',(1.1,-1.25565664448622,0.7));
#9110=CARTESIAN_POINT('',(1.1,-0.724814814814815,0.7));
#9111=CARTESIAN_POINT('',(1.10000000000005,-1.35674377243284,0.605845626926786));
#9112=CARTESIAN_POINT('Ctrl Pts',(1.09999997754868,-1.35674374570294,0.605845627052288));
#9113=CARTESIAN_POINT('Ctrl Pts',(1.09999999227748,-1.35627542940044,0.613744255356351));
#9114=CARTESIAN_POINT('Ctrl Pts',(1.1000044245081,-1.35483313756702,0.621542702113576));
#9115=CARTESIAN_POINT('Ctrl Pts',(1.10000632213307,-1.3525036790266,0.629082464357584));
#9116=CARTESIAN_POINT('Ctrl Pts',(1.1000073336739,-1.3512619466217,0.633101581650771));
#9117=CARTESIAN_POINT('Ctrl Pts',(1.10000777634458,-1.34976719347553,0.637047225321331));
#9118=CARTESIAN_POINT('Ctrl Pts',(1.10000752568741,-1.34802684471036,0.640893844816285));
#9119=CARTESIAN_POINT('Ctrl Pts',(1.10000705344834,-1.3447480208661,0.648140890909733));
#9120=CARTESIAN_POINT('Ctrl Pts',(1.10000374385205,-1.34063788586045,0.654954534019122));
#9121=CARTESIAN_POINT('Ctrl Pts',(1.10000230512149,-1.33576793982513,0.661175616324976));
#9122=CARTESIAN_POINT('Ctrl Pts',(1.10000200863552,-1.33476436716076,0.662457623989879));
#9123=CARTESIAN_POINT('Ctrl Pts',(1.10000181701501,-1.33372836971272,0.663714393476354));
#9124=CARTESIAN_POINT('Ctrl Pts',(1.10000180919237,-1.33266033853372,0.664944387472089));
#9125=CARTESIAN_POINT('Ctrl Pts',(1.10000179685332,-1.33097567746633,0.666884520904953));
#9126=CARTESIAN_POINT('Ctrl Pts',(1.10000223926429,-1.32921133126375,0.668758058859172));
#9127=CARTESIAN_POINT('Ctrl Pts',(1.10000288715521,-1.32737234926393,0.670562692084704));
#9128=CARTESIAN_POINT('Ctrl Pts',(1.10000489069569,-1.32168547392559,0.676143347135183));
#9129=CARTESIAN_POINT('Ctrl Pts',(1.10000845923633,-1.31535192007569,0.681005160308095));
#9130=CARTESIAN_POINT('Ctrl Pts',(1.1000097672184,-1.30853956043085,0.685101187995272));
#9131=CARTESIAN_POINT('Ctrl Pts',(1.10001062829021,-1.30405484229164,0.687797688271992));
#9132=CARTESIAN_POINT('Ctrl Pts',(1.10001067755751,-1.29936155475819,0.690161668140197));
#9133=CARTESIAN_POINT('Ctrl Pts',(1.10000992106221,-1.29450057597768,0.692169783635984));
#9134=CARTESIAN_POINT('Ctrl Pts',(1.10000876843985,-1.28709422081189,0.695229417764685));
#9135=CARTESIAN_POINT('Ctrl Pts',(1.100005676647,-1.27938091857402,0.69743146309387));
#9136=CARTESIAN_POINT('Ctrl Pts',(1.10000309801581,-1.2715114871423,0.698709794160748));
#9137=CARTESIAN_POINT('Ctrl Pts',(1.10000138449209,-1.26628217885177,0.699559256705032));
#9138=CARTESIAN_POINT('Ctrl Pts',(1.1,-1.26098326598685,0.700000000000001));
#9139=CARTESIAN_POINT('Ctrl Pts',(1.1,-1.25565664448621,0.7));
#9140=CARTESIAN_POINT('',(1.1,-1.39262953588351,0.));
#9141=CARTESIAN_POINT('Ctrl Pts',(1.1,-1.39262953588351,0.));
#9142=CARTESIAN_POINT('Ctrl Pts',(1.1,-1.38665944902278,0.100890429980357));
#9143=CARTESIAN_POINT('Ctrl Pts',(1.1,-1.38068638286488,0.201781712214768));
#9144=CARTESIAN_POINT('Ctrl Pts',(1.1,-1.36872453529477,0.403729561179669));
#9145=CARTESIAN_POINT('Ctrl Pts',(1.10000000000005,-1.3627356212621,0.504788200493074));
#9146=CARTESIAN_POINT('Ctrl Pts',(1.10000000000005,-1.35674377243284,0.605845626926786));
#9147=CARTESIAN_POINT('',(1.1,-1.44962962962963,0.));
#9148=CARTESIAN_POINT('Origin',(0.199725906950915,-1.4,-0.0104671912485888));
#9149=CARTESIAN_POINT('',(0.200274469199584,1.15262458915154,1.38777878078145E-17));
#9150=CARTESIAN_POINT('',(0.200274469199585,-0.7,0.));
#9151=CARTESIAN_POINT('',(0.231993417893744,1.12115139781563,0.605233595624295));
#9152=CARTESIAN_POINT('Ctrl Pts',(0.200274469199584,1.15262458915154,-5.50774703622636E-17));
#9153=CARTESIAN_POINT('Ctrl Pts',(0.210847451072758,1.1421331482829,0.201744512318911));
#9154=CARTESIAN_POINT('Ctrl Pts',(0.221420433966108,1.13164208276446,0.403489044103923));
#9155=CARTESIAN_POINT('Ctrl Pts',(0.231993417893744,1.12115139781563,0.605233595624295));
#9156=CARTESIAN_POINT('',(0.231993417893744,-1.12115139781563,0.605233595624295));
#9157=CARTESIAN_POINT('',(0.231993417893744,-0.7,0.605233595624295));
#9158=CARTESIAN_POINT('',(0.200274469199584,-1.15262458915154,1.38777878078145E-17));
#9159=CARTESIAN_POINT('Ctrl Pts',(0.231993417893744,-1.12115139781563,0.605233595624295));
#9160=CARTESIAN_POINT('Ctrl Pts',(0.221420433966108,-1.13164208276446,0.403489044103923));
#9161=CARTESIAN_POINT('Ctrl Pts',(0.210847451072758,-1.1421331482829,0.201744512318911));
#9162=CARTESIAN_POINT('Ctrl Pts',(0.200274469199584,-1.15262458915154,-6.67868538251071E-17));
#9163=CARTESIAN_POINT('',(0.200274469199585,-0.7,0.));
#9164=CARTESIAN_POINT('Origin',(6.07974599480623,0.,0.));
#9165=CARTESIAN_POINT('Ctrl Pts',(8.1,-1.69866351109718,4.37041895728907E-16));
#9166=CARTESIAN_POINT('Ctrl Pts',(8.9524267631348,-1.65897367198627,1.20944032620455E-7));
#9167=CARTESIAN_POINT('Ctrl Pts',(9.80407798130771,-1.59837060538327,2.76830114922109E-8));
#9168=CARTESIAN_POINT('Ctrl Pts',(10.6537697771985,-1.52488560579501,1.03413542584124E-8));
#9169=CARTESIAN_POINT('Ctrl Pts',(10.8359404901627,-1.50913069933138,6.62336842220622E-9));
#9170=CARTESIAN_POINT('Ctrl Pts',(11.0180211259896,-1.49278349820154,3.93228299510406E-9));
#9171=CARTESIAN_POINT('Ctrl Pts',(11.2000000002909,-1.47592264092474,-3.0227174540096E-11));
#9172=CARTESIAN_POINT('Ctrl Pts',(11.2000000002909,1.47592264092474,-3.02272213335841E-11));
#9173=CARTESIAN_POINT('Ctrl Pts',(10.4240589919717,1.54781576943643,1.68591524001238E-8));
#9174=CARTESIAN_POINT('Ctrl Pts',(9.64626799696257,1.61037563220813,6.17878738288937E-8));
#9175=CARTESIAN_POINT('Ctrl Pts',(8.86753211358286,1.65747704847969,5.27022751808308E-8));
#9176=CARTESIAN_POINT('Ctrl Pts',(8.61177933690776,1.67294611604661,4.97183789310355E-8));
#9177=CARTESIAN_POINT('Ctrl Pts',(8.35592462822135,1.68674740550612,3.63007687033005E-8));
#9178=CARTESIAN_POINT('Ctrl Pts',(8.1,1.69866351109718,3.71000138306103E-16));
#9179=CARTESIAN_POINT('',(7.9,1.70758761671949,0.));
#9180=CARTESIAN_POINT('',(7.9,1.7737037037037,0.));
#9181=CARTESIAN_POINT('Ctrl Pts',(7.90000000036908,1.70758761645525,-3.06814577203155E-11));
#9182=CARTESIAN_POINT('Ctrl Pts',(7.26247716501442,1.73478515342832,3.65175246633048E-8));
#9183=CARTESIAN_POINT('Ctrl Pts',(6.624575449312,1.74993328406844,-3.04558542439636E-7));
#9184=CARTESIAN_POINT('Ctrl Pts',(5.98677261990733,1.74972113442148,-3.1918790057331E-7));
#9185=CARTESIAN_POINT('Ctrl Pts',(5.35540610719671,1.74951112565922,-3.33669628155763E-7));
#9186=CARTESIAN_POINT('Ctrl Pts',(4.72663057529054,1.73425216511322,1.21151810208783E-7));
#9187=CARTESIAN_POINT('Ctrl Pts',(4.10000000045307,1.7011388979176,-4.27317258673188E-11));
#9188=CARTESIAN_POINT('',(3.9,1.68995649764597,0.));
#9189=CARTESIAN_POINT('',(3.9,1.7662962962963,0.));
#9190=CARTESIAN_POINT('Ctrl Pts',(3.9,1.68995649764597,-1.6113354923472E-17));
#9191=CARTESIAN_POINT('Ctrl Pts',(2.96252047830716,1.63464572816558,-1.61179993858831E-17));
#9192=CARTESIAN_POINT('Ctrl Pts',(2.02971500398675,1.53866944530133,-1.61823222708931E-17));
#9193=CARTESIAN_POINT('Ctrl Pts',(1.1,1.39262953588351,-1.60717230190728E-17));
#9194=CARTESIAN_POINT('',(0.9,1.3604297237941,0.));
#9195=CARTESIAN_POINT('',(0.9,1.44962962962963,0.));
#9196=CARTESIAN_POINT('',(0.28146619846596,1.25073018526678,0.));
#9197=CARTESIAN_POINT('Ctrl Pts',(0.899999999999963,1.36042972379409,2.53412200078296E-14));
#9198=CARTESIAN_POINT('Ctrl Pts',(0.693681964344164,1.32640030945436,-1.68820282978727E-7));
#9199=CARTESIAN_POINT('Ctrl Pts',(0.487510176034459,1.28986876146525,1.95094241611213E-11));
#9200=CARTESIAN_POINT('Ctrl Pts',(0.281466198465954,1.25073018526678,9.09211941846344E-16));
#9201=CARTESIAN_POINT('Ctrl Pts',(0.28146619846596,1.25073018526678,4.90059381963448E-17));
#9202=CARTESIAN_POINT('Ctrl Pts',(0.273672142824666,1.24924968434803,-1.60851827685828E-11));
#9203=CARTESIAN_POINT('Ctrl Pts',(0.266112037439191,1.2468180315926,-2.29735811958388E-6));
#9204=CARTESIAN_POINT('Ctrl Pts',(0.258922416881026,1.24354471831116,-3.39045428380668E-6));
#9205=CARTESIAN_POINT('Ctrl Pts',(0.254316658841251,1.24144779416325,-4.09070493067818E-6));
#9206=CARTESIAN_POINT('Ctrl Pts',(0.249862973385875,1.23900427835211,-4.3601744978078E-6));
#9207=CARTESIAN_POINT('Ctrl Pts',(0.245601965247185,1.23623285256398,-4.0505643599354E-6));
#9208=CARTESIAN_POINT('Ctrl Pts',(0.238945660500109,1.23190348870705,-3.5669089987193E-6));
#9209=CARTESIAN_POINT('Ctrl Pts',(0.232836306411817,1.22682685988243,-1.47564048465526E-6));
#9210=CARTESIAN_POINT('Ctrl Pts',(0.227416445112993,1.2210931256102,-3.43092614100725E-7));
#9211=CARTESIAN_POINT('Ctrl Pts',(0.225957664245637,1.21954986437275,-3.82620891408318E-8));
#9212=CARTESIAN_POINT('Ctrl Pts',(0.224549002474426,1.21795876469157,1.76022586487844E-7));
#9213=CARTESIAN_POINT('Ctrl Pts',(0.223193686986583,1.21632111005909,2.01577349231486E-7));
#9214=CARTESIAN_POINT('Ctrl Pts',(0.221344954485829,1.21408724984631,2.36435595047204E-7));
#9215=CARTESIAN_POINT('Ctrl Pts',(0.219595448227346,1.21176677459781,-7.7718209010198E-8));
#9216=CARTESIAN_POINT('Ctrl Pts',(0.217948412504407,1.20936721934621,-5.08402878561E-7));
#9217=CARTESIAN_POINT('Ctrl Pts',(0.213467776427723,1.20283941082417,-1.68004793834142E-6));
#9218=CARTESIAN_POINT('Ctrl Pts',(0.20978887558685,1.19579640990262,-3.43350901357988E-6));
#9219=CARTESIAN_POINT('Ctrl Pts',(0.206958221875648,1.18840352636746,-3.67425174897535E-6));
#9220=CARTESIAN_POINT('Ctrl Pts',(0.206193447398199,1.18640614723908,-3.7392946395744E-6));
#9221=CARTESIAN_POINT('Ctrl Pts',(0.205490847532167,1.18438308363371,-3.7149036306613E-6));
#9222=CARTESIAN_POINT('Ctrl Pts',(0.204851940804359,1.18233735619935,-3.6037364623937E-6));
#9223=CARTESIAN_POINT('Ctrl Pts',(0.202492508448082,1.17478264548698,-3.19320484275276E-6));
#9224=CARTESIAN_POINT('Ctrl Pts',(0.201019195184615,1.16698811697394,-1.36638523817118E-6));
#9225=CARTESIAN_POINT('Ctrl Pts',(0.200491965466086,1.15911075533121,-4.28455138775697E-7));
#9226=CARTESIAN_POINT('Ctrl Pts',(0.200347608840846,1.15695391685535,-1.71647870329038E-7));
#9227=CARTESIAN_POINT('Ctrl Pts',(0.200274469313241,1.15479080601565,-7.49035961899928E-12));
#9228=CARTESIAN_POINT('Ctrl Pts',(0.200274469199584,1.15262458915154,9.10729824887824E-18));
#9229=CARTESIAN_POINT('',(2.01407162049393E-18,1.15316892111334,2.77409355997279E-17));
#9230=CARTESIAN_POINT('',(0.,-1.4,0.));
#9231=CARTESIAN_POINT('',(0.243580684154574,1.44748675362873,2.77555756156289E-17));
#9232=CARTESIAN_POINT('Ctrl Pts',(0.243580684154575,1.44748675362873,-1.56125112837913E-16));
#9233=CARTESIAN_POINT('Ctrl Pts',(0.226022619058538,1.44415189332774,-6.74769223000006E-12));
#9234=CARTESIAN_POINT('Ctrl Pts',(0.208837776424359,1.43922483814223,-1.83343972289099E-6));
#9235=CARTESIAN_POINT('Ctrl Pts',(0.192216855517481,1.43283671850359,-2.37047811876899E-6));
#9236=CARTESIAN_POINT('Ctrl Pts',(0.175448307189507,1.42639185943196,-2.91228650265529E-6));
#9237=CARTESIAN_POINT('Ctrl Pts',(0.15925228528901,1.41845922211561,-2.09168970691363E-6));
#9238=CARTESIAN_POINT('Ctrl Pts',(0.143842215871583,1.4091253227419,-1.20497646612983E-7));
#9239=CARTESIAN_POINT('Ctrl Pts',(0.141154971457358,1.40749765525544,2.23243494969264E-7));
#9240=CARTESIAN_POINT('Ctrl Pts',(0.138491701959641,1.40582727297256,5.92673833856784E-7));
#9241=CARTESIAN_POINT('Ctrl Pts',(0.135853645420207,1.40411450883245,9.74556207071009E-7));
#9242=CARTESIAN_POINT('Ctrl Pts',(0.120686164410185,1.39426698768136,3.17018528370531E-6));
#9243=CARTESIAN_POINT('Ctrl Pts',(0.106484701177391,1.38310949089167,6.09567884445769E-6));
#9244=CARTESIAN_POINT('Ctrl Pts',(0.0934509959242968,1.37075049507673,5.10227143121889E-6));
#9245=CARTESIAN_POINT('Ctrl Pts',(0.0918301157095608,1.36921352217444,4.97873062758527E-6));
#9246=CARTESIAN_POINT('Ctrl Pts',(0.0902273306836925,1.36765791150105,4.78983320752683E-6));
#9247=CARTESIAN_POINT('Ctrl Pts',(0.0886430622088043,1.36608382581751,4.52250464763623E-6));
#9248=CARTESIAN_POINT('Ctrl Pts',(0.0755027622673366,1.35302798437193,2.30521792157715E-6));
#9249=CARTESIAN_POINT('Ctrl Pts',(0.0636322991078783,1.33870385142449,-4.95851449924696E-6));
#9250=CARTESIAN_POINT('Ctrl Pts',(0.0531272107863483,1.3233265665666,-1.07771754856876E-5));
#9251=CARTESIAN_POINT('Ctrl Pts',(0.0429100363670196,1.3083707283404,-1.64363639061758E-5));
#9252=CARTESIAN_POINT('Ctrl Pts',(0.0340657397255946,1.29253754778979,-2.07072841115287E-5));
#9253=CARTESIAN_POINT('Ctrl Pts',(0.026663056477648,1.27603964904139,-2.15377272154938E-5));
#9254=CARTESIAN_POINT('Ctrl Pts',(0.0217318501145713,1.26504977678014,-2.20909166714363E-5));
#9255=CARTESIAN_POINT('Ctrl Pts',(0.0174411483101006,1.25376411673155,-2.12025196266096E-5));
#9256=CARTESIAN_POINT('Ctrl Pts',(0.01382286588119,1.24224013948332,-1.91534441809703E-5));
#9257=CARTESIAN_POINT('Ctrl Pts',(0.00842668188255806,1.22505366970124,
-1.60975223868617E-5));
#9258=CARTESIAN_POINT('Ctrl Pts',(0.00456091079961661,1.20745571355567,
-1.03588883906395E-5));
#9259=CARTESIAN_POINT('Ctrl Pts',(0.0023097402764219,1.18964331095195,-5.71664032024866E-6));
#9260=CARTESIAN_POINT('Ctrl Pts',(0.00078319128522165,1.17756448131848,
-2.56866950429304E-6));
#9261=CARTESIAN_POINT('Ctrl Pts',(2.50028438421117E-9,1.16538650529032,
-1.91718613723104E-10));
#9262=CARTESIAN_POINT('Ctrl Pts',(-1.21430643318376E-17,1.15316892111333,
5.20417042793042E-18));
#9263=CARTESIAN_POINT('',(11.7295909468525,1.62672708026858,5.55111512312578E-17));
#9264=CARTESIAN_POINT('Ctrl Pts',(0.243580684154574,1.44748675362873,0.));
#9265=CARTESIAN_POINT('Ctrl Pts',(4.07225077172054,2.17467835246083,0.));
#9266=CARTESIAN_POINT('Ctrl Pts',(7.90092085928651,2.00057770191527,0.));
#9267=CARTESIAN_POINT('Ctrl Pts',(11.7295909468525,1.62672708026858,0.));
#9268=CARTESIAN_POINT('',(12.,1.32855945177638,-4.17473993839455E-17));
#9269=CARTESIAN_POINT('Ctrl Pts',(12.,1.32855945177638,2.42861286636753E-16));
#9270=CARTESIAN_POINT('Ctrl Pts',(11.9999999991614,1.34640852075174,-1.28298622986823E-11));
#9271=CARTESIAN_POINT('Ctrl Pts',(11.9983618543561,1.36418409382152,-2.22383001277967E-6));
#9272=CARTESIAN_POINT('Ctrl Pts',(11.9951861391139,1.38167870884165,-3.43465861540838E-6));
#9273=CARTESIAN_POINT('Ctrl Pts',(11.9919727904737,1.39938064150867,-4.65983598400874E-6));
#9274=CARTESIAN_POINT('Ctrl Pts',(11.9871848331028,1.41679645887758,-4.78742071954366E-6));
#9275=CARTESIAN_POINT('Ctrl Pts',(11.9808755917115,1.43370272794343,-3.5739118077222E-6));
#9276=CARTESIAN_POINT('Ctrl Pts',(11.9797611226834,1.43668906371449,-3.35955670324834E-6));
#9277=CARTESIAN_POINT('Ctrl Pts',(11.9785990681726,1.43965944485564,-3.11247275469786E-6));
#9278=CARTESIAN_POINT('Ctrl Pts',(11.9773895732386,1.44261255525912,-2.84353511336506E-6));
#9279=CARTESIAN_POINT('Ctrl Pts',(11.9705369081732,1.45934406518776,-1.31980853313606E-6));
#9280=CARTESIAN_POINT('Ctrl Pts',(11.9622259501015,1.47537448669426,1.24030492427686E-6));
#9281=CARTESIAN_POINT('Ctrl Pts',(11.9525330320198,1.49048867890869,8.79804099270529E-7));
#9282=CARTESIAN_POINT('Ctrl Pts',(11.9492586078121,1.49559449703792,7.58021100761347E-7));
#9283=CARTESIAN_POINT('Ctrl Pts',(11.9458260650319,1.50059560584699,2.73671093112169E-7));
#9284=CARTESIAN_POINT('Ctrl Pts',(11.9422371454499,1.50548309160802,-8.21070286398525E-7));
#9285=CARTESIAN_POINT('Ctrl Pts',(11.9335276940755,1.51734385321214,-3.47774636801117E-6));
#9286=CARTESIAN_POINT('Ctrl Pts',(11.923898315087,1.52853671512454,-9.61160164537397E-6));
#9287=CARTESIAN_POINT('Ctrl Pts',(11.9134480753511,1.53899918600446,-1.54908303532852E-5));
#9288=CARTESIAN_POINT('Ctrl Pts',(11.9006414429521,1.55182080751067,-2.26957483986032E-5));
#9289=CARTESIAN_POINT('Ctrl Pts',(11.8867118754531,1.56343792791748,-2.93307907620841E-5));
#9290=CARTESIAN_POINT('Ctrl Pts',(11.8718669715436,1.57375979462261,-3.2097080434168E-5));
#9291=CARTESIAN_POINT('Ctrl Pts',(11.8583226919989,1.58317731924447,-3.46210038525051E-5));
#9292=CARTESIAN_POINT('Ctrl Pts',(11.84401509256,1.59151672629289,-3.39892197405707E-5));
#9293=CARTESIAN_POINT('Ctrl Pts',(11.8290799708805,1.59867837245092,-3.04453078860132E-5));
#9294=CARTESIAN_POINT('Ctrl Pts',(11.8128282236205,1.60647136308226,-2.65889777530425E-5));
#9295=CARTESIAN_POINT('Ctrl Pts',(11.7959622791259,1.61280865470064,-1.93051308245346E-5));
#9296=CARTESIAN_POINT('Ctrl Pts',(11.7786680578171,1.61758555622507,-1.24065785496921E-5));
#9297=CARTESIAN_POINT('Ctrl Pts',(11.7626326571209,1.62201475420184,-6.0101616208217E-6));
#9298=CARTESIAN_POINT('Ctrl Pts',(11.7462278952123,1.62510256303752,-1.15598952599692E-10));
#9299=CARTESIAN_POINT('Ctrl Pts',(11.7295909468525,1.62672708026857,-1.01481323344643E-16));
#9300=CARTESIAN_POINT('',(12.,-1.32855945177638,-2.7831599589297E-17));
#9301=CARTESIAN_POINT('',(12.,1.6,0.));
#9302=CARTESIAN_POINT('',(11.7295909468525,-1.62672708026858,-2.77555756156289E-17));
#9303=CARTESIAN_POINT('Ctrl Pts',(11.7295909468525,-1.62672708026858,2.76688394418301E-16));
#9304=CARTESIAN_POINT('Ctrl Pts',(11.7473502233519,-1.62499297457843,3.63491969896433E-13));
#9305=CARTESIAN_POINT('Ctrl Pts',(11.7648769397846,-1.62163540491215,-2.46542030701863E-6));
#9306=CARTESIAN_POINT('Ctrl Pts',(11.7819744899096,-1.61677476461769,-3.87870576098494E-6));
#9307=CARTESIAN_POINT('Ctrl Pts',(11.799277951102,-1.61185558613358,-5.30901184740094E-6));
#9308=CARTESIAN_POINT('Ctrl Pts',(11.8161433440738,-1.60539638769883,-5.61072687595782E-6));
#9309=CARTESIAN_POINT('Ctrl Pts',(11.8323535184498,-1.59747214364331,-4.43708131311936E-6));
#9310=CARTESIAN_POINT('Ctrl Pts',(11.8351986841263,-1.59608130189932,-4.23108623901291E-6));
#9311=CARTESIAN_POINT('Ctrl Pts',(11.8380235988884,-1.59464521634493,-3.98890160078043E-6));
#9312=CARTESIAN_POINT('Ctrl Pts',(11.8408269920241,-1.59316415515964,-3.72087260345577E-6));
#9313=CARTESIAN_POINT('Ctrl Pts',(11.8568148563263,-1.58471760338924,-2.19229240409177E-6));
#9314=CARTESIAN_POINT('Ctrl Pts',(11.8719627312575,-1.57488689795395,5.08047814114288E-7));
#9315=CARTESIAN_POINT('Ctrl Pts',(11.8860639991294,-1.56376935451958,3.7910357452838E-7));
#9316=CARTESIAN_POINT('Ctrl Pts',(11.8908390360804,-1.5600046802233,3.35439876042474E-7));
#9317=CARTESIAN_POINT('Ctrl Pts',(11.8954938739134,-1.55609205312677,-6.31409548673105E-8));
#9318=CARTESIAN_POINT('Ctrl Pts',(11.9000197537765,-1.55203410647271,-1.07033715310124E-6));
#9319=CARTESIAN_POINT('Ctrl Pts',(11.9109521284419,-1.54223203603875,-3.50324446252274E-6));
#9320=CARTESIAN_POINT('Ctrl Pts',(11.9211333865357,-1.53158293117673,-9.37257606292525E-6));
#9321=CARTESIAN_POINT('Ctrl Pts',(11.9305114837192,-1.52019095639426,-1.50133174764804E-5));
#9322=CARTESIAN_POINT('Ctrl Pts',(11.9420285825687,-1.50620064502377,-2.19406264148308E-5));
#9323=CARTESIAN_POINT('Ctrl Pts',(11.9522379825693,-1.49120969914507,-2.8349487615449E-5));
#9324=CARTESIAN_POINT('Ctrl Pts',(11.9610699533786,-1.47543375940277,-3.10096306454085E-5));
#9325=CARTESIAN_POINT('Ctrl Pts',(11.9691383866925,-1.46102167397773,-3.34398002084833E-5));
#9326=CARTESIAN_POINT('Ctrl Pts',(11.976057247492,-1.44595309822982,-3.28127654573608E-5));
#9327=CARTESIAN_POINT('Ctrl Pts',(11.9817405815488,-1.43037347552767,-2.93737351251587E-5));
#9328=CARTESIAN_POINT('Ctrl Pts',(11.9879190063177,-1.41343666945002,-2.56351214921306E-5));
#9329=CARTESIAN_POINT('Ctrl Pts',(11.9925890154887,-1.39602986621001,-1.86015881889918E-5));
#9330=CARTESIAN_POINT('Ctrl Pts',(11.9956646601292,-1.37834843064327,-1.1951505214167E-5));
#9331=CARTESIAN_POINT('Ctrl Pts',(11.9985188379205,-1.36194017591583,-5.78027239782095E-6));
#9332=CARTESIAN_POINT('Ctrl Pts',(11.9999999979315,-1.34529424449622,-1.63143103698095E-10));
#9333=CARTESIAN_POINT('Ctrl Pts',(12.,-1.32855945177638,6.07153216591882E-17));
#9334=CARTESIAN_POINT('',(0.243580684154574,-1.44748675362873,-2.77555756156289E-17));
#9335=CARTESIAN_POINT('Ctrl Pts',(11.7295909468525,-1.62672708026858,0.));
#9336=CARTESIAN_POINT('Ctrl Pts',(7.90092085928651,-2.00057770191527,0.));
#9337=CARTESIAN_POINT('Ctrl Pts',(4.07225077172054,-2.17467835246083,0.));
#9338=CARTESIAN_POINT('Ctrl Pts',(0.243580684154574,-1.44748675362873,0.));
#9339=CARTESIAN_POINT('',(-2.01407162049393E-18,-1.15316892111334,-2.77409355997279E-17));
#9340=CARTESIAN_POINT('Ctrl Pts',(-1.45716771982052E-16,-1.15316892111333,
-8.67361737988404E-17));
#9341=CARTESIAN_POINT('Ctrl Pts',(1.25998894435939E-9,-1.17105087373522,
-1.90287520688926E-11));
#9342=CARTESIAN_POINT('Ctrl Pts',(0.00163339464743996,-1.18886359576077,
-1.42965894531121E-6));
#9343=CARTESIAN_POINT('Ctrl Pts',(0.00480727841906161,-1.20639511031145,
-1.64093682142839E-6));
#9344=CARTESIAN_POINT('Ctrl Pts',(0.00800796397580062,-1.22407466931478,
-1.8539988284852E-6));
#9345=CARTESIAN_POINT('Ctrl Pts',(0.0127756311263789,-1.24146980201313,
-7.66483898132055E-7));
#9346=CARTESIAN_POINT('Ctrl Pts',(0.0190655400899108,-1.25835467436912,
1.24978183846727E-6));
#9347=CARTESIAN_POINT('Ctrl Pts',(0.0201762582672253,-1.26133632875492,
1.60582880463507E-6));
#9348=CARTESIAN_POINT('Ctrl Pts',(0.0213345630164365,-1.2643020159517,1.98173645466097E-6));
#9349=CARTESIAN_POINT('Ctrl Pts',(0.022540357064946,-1.26725040777374,2.36324320385681E-6));
#9350=CARTESIAN_POINT('Ctrl Pts',(0.0293845669280623,-1.28398578013164,
4.5287143794027E-6));
#9351=CARTESIAN_POINT('Ctrl Pts',(0.0376942987862453,-1.30001720705818,
7.20349268724091E-6));
#9352=CARTESIAN_POINT('Ctrl Pts',(0.0474014865253391,-1.31512615530125,
5.82569015349308E-6));
#9353=CARTESIAN_POINT('Ctrl Pts',(0.0485928463173857,-1.31698047129067,
5.65659292531477E-6));
#9354=CARTESIAN_POINT('Ctrl Pts',(0.049805315173965,-1.3188208685659,5.4220814195758E-6));
#9355=CARTESIAN_POINT('Ctrl Pts',(0.0510388164126442,-1.32064691964073,
5.10992468070797E-6));
#9356=CARTESIAN_POINT('Ctrl Pts',(0.0614399911345998,-1.33604461498541,
2.47774509321499E-6));
#9357=CARTESIAN_POINT('Ctrl Pts',(0.0733332132114129,-1.35042574344132,
-5.3152380038924E-6));
#9358=CARTESIAN_POINT('Ctrl Pts',(0.0865238753361435,-1.36365441213776,
-1.1550981620978E-5));
#9359=CARTESIAN_POINT('Ctrl Pts',(0.0993129767592984,-1.37648036310613,
-1.75968917362996E-5));
#9360=CARTESIAN_POINT('Ctrl Pts',(0.113220041589059,-1.38812080263946,-2.21381304374214E-5));
#9361=CARTESIAN_POINT('Ctrl Pts',(0.128049501721596,-1.3984678073416,-2.30260298918279E-5));
#9362=CARTESIAN_POINT('Ctrl Pts',(0.137898881094142,-1.40534004502052,-2.36157518704412E-5));
#9363=CARTESIAN_POINT('Ctrl Pts',(0.148156110210342,-1.41164106947418,-2.26770903305374E-5));
#9364=CARTESIAN_POINT('Ctrl Pts',(0.158771208267938,-1.41732893485082,-2.05010084084185E-5));
#9365=CARTESIAN_POINT('Ctrl Pts',(0.174640735071984,-1.42583226958806,-1.72477751171679E-5));
#9366=CARTESIAN_POINT('Ctrl Pts',(0.191199787345415,-1.4329086754137,-1.11085100333009E-5));
#9367=CARTESIAN_POINT('Ctrl Pts',(0.208270835533445,-1.43843835369108,-6.12965879291162E-6));
#9368=CARTESIAN_POINT('Ctrl Pts',(0.219822542278978,-1.44218019901621,-2.76054936125183E-6));
#9369=CARTESIAN_POINT('Ctrl Pts',(0.231609382520684,-1.4452130041726,-1.10646384277296E-10));
#9370=CARTESIAN_POINT('Ctrl Pts',(0.243580684154575,-1.44748675362873,-8.67361737988404E-18));
#9371=CARTESIAN_POINT('',(0.,-1.4,0.));
#9372=CARTESIAN_POINT('',(0.28146619846596,-1.25073018526678,-1.38777878078145E-17));
#9373=CARTESIAN_POINT('Ctrl Pts',(0.200274469199584,-1.15262458915154,-4.38017677684144E-17));
#9374=CARTESIAN_POINT('Ctrl Pts',(0.200274469606231,-1.16056122076396,-2.67994619525583E-11));
#9375=CARTESIAN_POINT('Ctrl Pts',(0.201251993787099,-1.16844573575355,-2.06906772440415E-6));
#9376=CARTESIAN_POINT('Ctrl Pts',(0.203125250303271,-1.17612349127761,-3.03593176598444E-6));
#9377=CARTESIAN_POINT('Ctrl Pts',(0.204328175564463,-1.18105381768481,-3.65681052429326E-6));
#9378=CARTESIAN_POINT('Ctrl Pts',(0.205901645655995,-1.18589907428975,-3.87486521964464E-6));
#9379=CARTESIAN_POINT('Ctrl Pts',(0.207834893326199,-1.19061551412018,-3.56660141708203E-6));
#9380=CARTESIAN_POINT('Ctrl Pts',(0.210845733886816,-1.19796089907112,-3.08651126907409E-6));
#9381=CARTESIAN_POINT('Ctrl Pts',(0.214691665920849,-1.20490884791767,-1.13290501265697E-6));
#9382=CARTESIAN_POINT('Ctrl Pts',(0.219311372289421,-1.21130241743461,-1.88024479619773E-7));
#9383=CARTESIAN_POINT('Ctrl Pts',(0.220549822002528,-1.21301640393121,6.52788543367939E-8));
#9384=CARTESIAN_POINT('Ctrl Pts',(0.22184414018537,-1.21469042595737,2.26073670777299E-7));
#9385=CARTESIAN_POINT('Ctrl Pts',(0.223193686901845,-1.21632111014354,1.99977909429435E-7));
#9386=CARTESIAN_POINT('Ctrl Pts',(0.225054776233359,-1.21856990146355,1.63990609064731E-7));
#9387=CARTESIAN_POINT('Ctrl Pts',(0.227020882846909,-1.2207363067163,-2.2494482424301E-7));
#9388=CARTESIAN_POINT('Ctrl Pts',(0.229085096241527,-1.22281561536867,-7.25033596408456E-7));
#9389=CARTESIAN_POINT('Ctrl Pts',(0.234663732853057,-1.22843504764494,-2.07654770860772E-6));
#9390=CARTESIAN_POINT('Ctrl Pts',(0.240898147116973,-1.23336261820331,-3.93931381885212E-6));
#9391=CARTESIAN_POINT('Ctrl Pts',(0.247634917667946,-1.2375211924479,-4.15647360184107E-6));
#9392=CARTESIAN_POINT('Ctrl Pts',(0.24944409362824,-1.23863798757926,-4.21479238469909E-6));
#9393=CARTESIAN_POINT('Ctrl Pts',(0.251289686356224,-1.23969909864123,-4.17584617698396E-6));
#9394=CARTESIAN_POINT('Ctrl Pts',(0.253169062337335,-1.24070249413235,-4.04352721072409E-6));
#9395=CARTESIAN_POINT('Ctrl Pts',(0.260147540238377,-1.24442829106235,-3.55220190316667E-6));
#9396=CARTESIAN_POINT('Ctrl Pts',(0.267526846148503,-1.24732811138375,-1.51439637010182E-6));
#9397=CARTESIAN_POINT('Ctrl Pts',(0.275164162321015,-1.24931347733136,-4.73394739174148E-7));
#9398=CARTESIAN_POINT('Ctrl Pts',(0.277246452424842,-1.24985478107889,-1.89568936341825E-7));
#9399=CARTESIAN_POINT('Ctrl Pts',(0.27934803608603,-1.25032783487679,-4.20368826828312E-12));
#9400=CARTESIAN_POINT('Ctrl Pts',(0.28146619846596,-1.25073018526678,1.2793585635329E-17));
#9401=CARTESIAN_POINT('',(0.9,-1.3604297237941,0.));
#9402=CARTESIAN_POINT('Ctrl Pts',(0.281466198465954,-1.25073018526678,9.63150999927498E-16));
#9403=CARTESIAN_POINT('Ctrl Pts',(0.487510152792939,-1.28986875705046,1.95065110193295E-11));
#9404=CARTESIAN_POINT('Ctrl Pts',(0.693681940810289,-1.32640030557063,-1.68784634270162E-7));
#9405=CARTESIAN_POINT('Ctrl Pts',(0.899999999999961,-1.36042972379409,2.52314774976951E-14));
#9406=CARTESIAN_POINT('',(0.9,1.44962962962963,0.));
#9407=CARTESIAN_POINT('',(3.9,-1.68995649764597,0.));
#9408=CARTESIAN_POINT('Ctrl Pts',(1.1,-1.39262953588351,-2.05019623674552E-17));
#9409=CARTESIAN_POINT('Ctrl Pts',(2.02971449277185,-1.53866936499954,-2.04062575199768E-17));
#9410=CARTESIAN_POINT('Ctrl Pts',(2.96251993741879,-1.63464569625347,-2.05230086706555E-17));
#9411=CARTESIAN_POINT('Ctrl Pts',(3.9,-1.68995649764597,-2.05203881127908E-17));
#9412=CARTESIAN_POINT('',(3.9,1.7662962962963,0.));
#9413=CARTESIAN_POINT('',(7.9,-1.70758761671949,0.));
#9414=CARTESIAN_POINT('Ctrl Pts',(4.10000000045307,-1.7011388979176,-4.27317380631109E-11));
#9415=CARTESIAN_POINT('Ctrl Pts',(4.72643887491804,-1.7342420350347,1.20853286712337E-7));
#9416=CARTESIAN_POINT('Ctrl Pts',(5.35502164560988,-1.74950180199062,-3.33551248611792E-7));
#9417=CARTESIAN_POINT('Ctrl Pts',(5.98619394951577,-1.74972093772735,-3.1920111515717E-7));
#9418=CARTESIAN_POINT('Ctrl Pts',(6.62418968669829,-1.74994244248134,-3.0469584628258E-7));
#9419=CARTESIAN_POINT('Ctrl Pts',(7.26228442347589,-1.73479337602516,3.6583895104054E-8));
#9420=CARTESIAN_POINT('Ctrl Pts',(7.90000000036908,-1.70758761645525,-3.06816097140251E-11));
#9421=CARTESIAN_POINT('',(7.9,1.7737037037037,0.));
#9422=CARTESIAN_POINT('',(11.4,-1.45718524058191,0.));
#9423=CARTESIAN_POINT('',(11.7095901160181,-1.42740242188993,1.38777878078145E-17));
#9424=CARTESIAN_POINT('Ctrl Pts',(11.4000000008084,-1.45718524050535,1.02728155843002E-16));
#9425=CARTESIAN_POINT('Ctrl Pts',(11.5032315878449,-1.44740895658952,-1.62414911853346E-10));
#9426=CARTESIAN_POINT('Ctrl Pts',(11.6064290066394,-1.43747657129068,3.17212713797596E-13));
#9427=CARTESIAN_POINT('Ctrl Pts',(11.7095901160181,-1.42740242188993,-1.31135713082882E-16));
#9428=CARTESIAN_POINT('',(11.7997255308004,-1.32801330383774,0.));
#9429=CARTESIAN_POINT('Ctrl Pts',(11.7095901160181,-1.42740242188993,-9.19403442267708E-17));
#9430=CARTESIAN_POINT('Ctrl Pts',(11.7174875668098,-1.42663119997609,-1.06723531187443E-12));
#9431=CARTESIAN_POINT('Ctrl Pts',(11.7252481284326,-1.42489860698852,-1.31351091787008E-6));
#9432=CARTESIAN_POINT('Ctrl Pts',(11.7327147629935,-1.4222933789697,-1.57347087725304E-6));
#9433=CARTESIAN_POINT('Ctrl Pts',(11.7375034508718,-1.42062252930751,-1.7401948673154E-6));
#9434=CARTESIAN_POINT('Ctrl Pts',(11.742171336984,-1.41859157258352,-1.52962160850981E-6));
#9435=CARTESIAN_POINT('Ctrl Pts',(11.7466731630754,-1.4162133745499,-1.06822103866601E-6));
#9436=CARTESIAN_POINT('Ctrl Pts',(11.7538080604269,-1.41244419322064,-3.36952074275293E-7));
#9437=CARTESIAN_POINT('Ctrl Pts',(11.7604421378066,-1.40785009750528,1.23525126371337E-6));
#9438=CARTESIAN_POINT('Ctrl Pts',(11.7664060685299,-1.40250292630552,-7.85770423176645E-8));
#9439=CARTESIAN_POINT('Ctrl Pts',(11.7700505374369,-1.39923534992309,-8.81437879006801E-7));
#9440=CARTESIAN_POINT('Ctrl Pts',(11.7734443324447,-1.39568546479044,-2.84121358692309E-6));
#9441=CARTESIAN_POINT('Ctrl Pts',(11.7765701913309,-1.39188797822873,-4.73246891796253E-6));
#9442=CARTESIAN_POINT('Ctrl Pts',(11.7816218974528,-1.38575085342217,-7.78893003218221E-6));
#9443=CARTESIAN_POINT('Ctrl Pts',(11.7859196635778,-1.3790373064984,-1.04294718165207E-5));
#9444=CARTESIAN_POINT('Ctrl Pts',(11.7894058487846,-1.37190723377291,-1.0649753115785E-5));
#9445=CARTESIAN_POINT('Ctrl Pts',(11.7909886780302,-1.36866997385604,-1.07497672177443E-5));
#9446=CARTESIAN_POINT('Ctrl Pts',(11.7924036476919,-1.36534638272796,-1.04045251440782E-5));
#9447=CARTESIAN_POINT('Ctrl Pts',(11.7936422141268,-1.36194984358789,-9.67400732978531E-6));
#9448=CARTESIAN_POINT('Ctrl Pts',(11.7963517531347,-1.35451943450186,-8.0758964348484E-6));
#9449=CARTESIAN_POINT('Ctrl Pts',(11.7981920551596,-1.34681816044402,-4.45435127417515E-6));
#9450=CARTESIAN_POINT('Ctrl Pts',(11.7990923524223,-1.33899256731255,-1.99131993767782E-6));
#9451=CARTESIAN_POINT('Ctrl Pts',(11.7995108157868,-1.33535518645399,-8.46488755312323E-7));
#9452=CARTESIAN_POINT('Ctrl Pts',(11.7997255306472,-1.33169069466208,-1.20180646731727E-11));
#9453=CARTESIAN_POINT('Ctrl Pts',(11.7997255308004,-1.32801330383774,1.56125112837913E-17));
#9454=CARTESIAN_POINT('',(11.7997255308004,1.32801330383774,-1.38777878078145E-17));
#9455=CARTESIAN_POINT('',(11.7997255308004,0.8,0.));
#9456=CARTESIAN_POINT('',(11.7095901160181,1.42740242188993,1.38777878078145E-17));
#9457=CARTESIAN_POINT('Ctrl Pts',(11.7997255308004,1.32801330383774,3.29597460435593E-17));
#9458=CARTESIAN_POINT('Ctrl Pts',(11.7997255306701,1.33594993357028,-3.19998942079111E-12));
#9459=CARTESIAN_POINT('Ctrl Pts',(11.7987557313351,1.34384388324515,-1.1738056914779E-6));
#9460=CARTESIAN_POINT('Ctrl Pts',(11.7968890528831,1.35153020534854,-1.35082478761126E-6));
#9461=CARTESIAN_POINT('Ctrl Pts',(11.7956902940742,1.35646627043222,-1.46450435604653E-6));
#9462=CARTESIAN_POINT('Ctrl Pts',(11.7941204989552,1.36131691981906,-1.21679535622301E-6));
#9463=CARTESIAN_POINT('Ctrl Pts',(11.7921880664813,1.36603565236267,-7.51718013047842E-7));
#9464=CARTESIAN_POINT('Ctrl Pts',(11.7891321441143,1.37349779167052,-1.62510435539431E-8));
#9465=CARTESIAN_POINT('Ctrl Pts',(11.7852081688769,1.38054242009704,1.47305143123643E-6));
#9466=CARTESIAN_POINT('Ctrl Pts',(11.7804707482717,1.38699431162271,4.31295153147674E-8));
#9467=CARTESIAN_POINT('Ctrl Pts',(11.7775673564694,1.39094843993989,-8.33217322910001E-7));
#9468=CARTESIAN_POINT('Ctrl Pts',(11.774357304366,1.39467961749964,-2.88177890715362E-6));
#9469=CARTESIAN_POINT('Ctrl Pts',(11.7708736118052,1.39816709864095,-4.85419454747415E-6));
#9470=CARTESIAN_POINT('Ctrl Pts',(11.7652557092992,1.40379111072049,-8.03496856102318E-6));
#9471=CARTESIAN_POINT('Ctrl Pts',(11.7589908599241,1.40872063947841,-1.07717451179728E-5));
#9472=CARTESIAN_POINT('Ctrl Pts',(11.7522324303862,1.41288246393566,-1.10093962897399E-5));
#9473=CARTESIAN_POINT('Ctrl Pts',(11.7491699691574,1.41476832010531,-1.11170836593312E-5));
#9474=CARTESIAN_POINT('Ctrl Pts',(11.7460056456443,1.41649603445901,-1.07652933077188E-5));
#9475=CARTESIAN_POINT('Ctrl Pts',(11.7427518690514,1.41805582819498,-1.00150721194158E-5));
#9476=CARTESIAN_POINT('Ctrl Pts',(11.7356218627913,1.421473806899,-8.37111113549047E-6));
#9477=CARTESIAN_POINT('Ctrl Pts',(11.7281378774234,1.42405291512428,-4.62166314666036E-6));
#9478=CARTESIAN_POINT('Ctrl Pts',(11.7204387731059,1.42570834923663,-2.06587013620581E-6));
#9479=CARTESIAN_POINT('Ctrl Pts',(11.7168648812537,1.42647679479109,-8.79481766934018E-7));
#9480=CARTESIAN_POINT('Ctrl Pts',(11.7132443218769,1.42704557200794,-8.45784208685192E-12));
#9481=CARTESIAN_POINT('Ctrl Pts',(11.7095901160181,1.42740242188993,2.53703308361608E-17));
#9482=CARTESIAN_POINT('',(11.4,1.45718524058191,0.));
#9483=CARTESIAN_POINT('Ctrl Pts',(11.7095901160181,1.42740242188993,-2.09644042577228E-16));
#9484=CARTESIAN_POINT('Ctrl Pts',(11.6064290073882,1.43747657121756,3.16925904777201E-13));
#9485=CARTESIAN_POINT('Ctrl Pts',(11.5032315885351,1.44740895652415,-1.62368751268212E-10));
#9486=CARTESIAN_POINT('Ctrl Pts',(11.4000000008083,1.45718524050537,-7.57963810214684E-17));
#9487=CARTESIAN_POINT('',(11.4,-1.53779953703704,0.));
#9488=CARTESIAN_POINT('Origin',(10.,0.,0.));
#9489=CARTESIAN_POINT('',(9.6,-4.89858719658942E-17,0.7));
#9490=CARTESIAN_POINT('Origin',(10.,0.,0.7));
#9491=CARTESIAN_POINT('',(9.6,-4.89858719658942E-17,0.));
#9492=CARTESIAN_POINT('Origin',(2.,0.,0.));
#9493=CARTESIAN_POINT('',(1.6,-4.89858719658941E-17,0.7));
#9494=CARTESIAN_POINT('Origin',(2.,0.,0.7));
#9495=CARTESIAN_POINT('',(1.6,-4.89858719658941E-17,0.));
#9496=CARTESIAN_POINT('Origin',(11.4,-1.53779953703704,0.));
#9497=CARTESIAN_POINT('',(11.4,-1.4227102204299,0.605660349289938));
#9498=CARTESIAN_POINT('Ctrl Pts',(11.4,-1.45718524058191,0.));
#9499=CARTESIAN_POINT('Ctrl Pts',(11.4,-1.45144762186897,0.100853500740053));
#9500=CARTESIAN_POINT('Ctrl Pts',(11.4,-1.44570843451869,0.201707502489292));
#9501=CARTESIAN_POINT('Ctrl Pts',(11.4,-1.43421679834229,0.403593890565801));
#9502=CARTESIAN_POINT('Ctrl Pts',(11.4,-1.42846427656079,0.504627461196798));
#9503=CARTESIAN_POINT('Ctrl Pts',(11.4,-1.4227102204299,0.605660349289938));
#9504=CARTESIAN_POINT('',(11.4,1.4227102204299,0.605660349289938));
#9505=CARTESIAN_POINT('Ctrl Pts',(11.4,1.4227102204299,0.605660349289938));
#9506=CARTESIAN_POINT('Ctrl Pts',(11.4,1.42846501637408,0.504614471147338));
#9507=CARTESIAN_POINT('Ctrl Pts',(11.4,1.43421827757761,0.403567910233218));
#9508=CARTESIAN_POINT('Ctrl Pts',(11.4,1.44570991295315,0.201681522149997));
#9509=CARTESIAN_POINT('Ctrl Pts',(11.4,1.45144836088146,0.100840510682596));
#9510=CARTESIAN_POINT('Ctrl Pts',(11.4,1.45718524058191,0.));
#9511=CARTESIAN_POINT('',(11.4,1.32241589772268,0.7));
#9512=CARTESIAN_POINT('Ctrl Pts',(11.3999999999682,1.32241589773435,0.7));
#9513=CARTESIAN_POINT('Ctrl Pts',(11.4000000023735,1.33035873561384,0.69999999792071));
#9514=CARTESIAN_POINT('Ctrl Pts',(11.3999980827719,1.33823923135401,0.699006238562837));
#9515=CARTESIAN_POINT('Ctrl Pts',(11.3999964146773,1.34591623266897,0.697118452648154));
#9516=CARTESIAN_POINT('Ctrl Pts',(11.3999954805754,1.35021521026861,0.696061327733467));
#9517=CARTESIAN_POINT('Ctrl Pts',(11.3999946303028,1.35445042327231,0.694722827332644));
#9518=CARTESIAN_POINT('Ctrl Pts',(11.3999940855437,1.35859537550353,0.6931136259882));
#9519=CARTESIAN_POINT('Ctrl Pts',(11.3999931076272,1.36603612757745,0.690224891070856));
#9520=CARTESIAN_POINT('Ctrl Pts',(11.3999932937992,1.3731074395729,0.686497549823264));
#9521=CARTESIAN_POINT('Ctrl Pts',(11.3999945206258,1.37966241828116,0.682010734965951));
#9522=CARTESIAN_POINT('Ctrl Pts',(11.3999951957832,1.38326980879772,0.679541513617388));
#9523=CARTESIAN_POINT('Ctrl Pts',(11.399996159718,1.38672054258633,0.67684140394947));
#9524=CARTESIAN_POINT('Ctrl Pts',(11.3999970106794,1.38998612808193,0.67391813047908));
#9525=CARTESIAN_POINT('Ctrl Pts',(11.399997834674,1.39314822810011,0.671087494715186));
#9526=CARTESIAN_POINT('Ctrl Pts',(11.3999985616145,1.39611771109305,0.668064564866167));
#9527=CARTESIAN_POINT('Ctrl Pts',(11.3999985600482,1.39887227052748,0.664860274403491));
#9528=CARTESIAN_POINT('Ctrl Pts',(11.3999985571253,1.40401282028653,0.65888043807832));
#9529=CARTESIAN_POINT('Ctrl Pts',(11.3999962993541,1.40840780441339,0.652270325570232));
#9530=CARTESIAN_POINT('Ctrl Pts',(11.399995545677,1.411994629421,0.6451936465425));
#9531=CARTESIAN_POINT('Ctrl Pts',(11.3999954685939,1.41236147527551,0.644469872631166));
#9532=CARTESIAN_POINT('Ctrl Pts',(11.3999954033687,1.41271982702329,0.643741199273148));
#9533=CARTESIAN_POINT('Ctrl Pts',(11.399995351278,1.41306958904162,0.643007791034547));
#9534=CARTESIAN_POINT('Ctrl Pts',(11.3999948427782,1.41648390439843,0.635848388696429));
#9535=CARTESIAN_POINT('Ctrl Pts',(11.3999960181446,1.41904356023948,0.628323447569199));
#9536=CARTESIAN_POINT('Ctrl Pts',(11.3999977140636,1.42069349507095,0.620600117586001));
#9537=CARTESIAN_POINT('Ctrl Pts',(11.3999987928026,1.4217429844709,0.615687467222433));
#9538=CARTESIAN_POINT('Ctrl Pts',(11.4,1.42242354791745,0.610693903223035));
#9539=CARTESIAN_POINT('Ctrl Pts',(11.4,1.42271022042989,0.605660349289938));
#9540=CARTESIAN_POINT('',(11.4,-1.32241589772233,0.7));
#9541=CARTESIAN_POINT('',(11.4,-0.768899768518519,0.7));
#9542=CARTESIAN_POINT('Ctrl Pts',(11.4,-1.4227102204299,0.605660349289938));
#9543=CARTESIAN_POINT('Ctrl Pts',(11.4,-1.42225988230954,0.613567634148305));
#9544=CARTESIAN_POINT('Ctrl Pts',(11.399997277834,-1.42084002197897,0.621378952482038));
#9545=CARTESIAN_POINT('Ctrl Pts',(11.3999960666067,-1.41853584574224,0.62893480307212));
#9546=CARTESIAN_POINT('Ctrl Pts',(11.3999954054252,-1.41727804822547,0.633059370437125));
#9547=CARTESIAN_POINT('Ctrl Pts',(11.399995101512,-1.41575577202439,0.637107840337094));
#9548=CARTESIAN_POINT('Ctrl Pts',(11.3999952458732,-1.4139766528271,0.641052464558972));
#9549=CARTESIAN_POINT('Ctrl Pts',(11.3999955106959,-1.41071295596475,0.648288661951321));
#9550=CARTESIAN_POINT('Ctrl Pts',(11.3999975070228,-1.40662392062869,0.655096264526915));
#9551=CARTESIAN_POINT('Ctrl Pts',(11.3999983091255,-1.40177626405188,0.661313589686923));
#9552=CARTESIAN_POINT('Ctrl Pts',(11.3999984645713,-1.40083679843637,0.66251849418371));
#9553=CARTESIAN_POINT('Ctrl Pts',(11.3999985618942,-1.3998687022723,0.663701157110503));
#9554=CARTESIAN_POINT('Ctrl Pts',(11.3999985615247,-1.39887227038638,0.664860274403572));
#9555=CARTESIAN_POINT('Ctrl Pts',(11.3999985608543,-1.39706426040285,0.666963474499402));
#9556=CARTESIAN_POINT('Ctrl Pts',(11.3999982409398,-1.39516298427334,0.668989190735049));
#9557=CARTESIAN_POINT('Ctrl Pts',(11.3999977953094,-1.39317470503404,0.670934323115149));
#9558=CARTESIAN_POINT('Ctrl Pts',(11.3999965209597,-1.38748891009577,0.67649673287249));
#9559=CARTESIAN_POINT('Ctrl Pts',(11.3999944455422,-1.38115857071774,0.681340422576046));
#9560=CARTESIAN_POINT('Ctrl Pts',(11.3999937508435,-1.37434881732181,0.685413525744465));
#9561=CARTESIAN_POINT('Ctrl Pts',(11.3999933041982,-1.36997059693002,0.688032261301096));
#9562=CARTESIAN_POINT('Ctrl Pts',(11.3999933336943,-1.3653932120823,0.69033179581025));
#9563=CARTESIAN_POINT('Ctrl Pts',(11.399993839827,-1.36065445462682,0.69228884175444));
#9564=CARTESIAN_POINT('Ctrl Pts',(11.3999946245508,-1.35330733883187,0.695323106179894));
#9565=CARTESIAN_POINT('Ctrl Pts',(11.3999965692242,-1.34565642326237,0.69750197024776));
#9566=CARTESIAN_POINT('Ctrl Pts',(11.3999981510416,-1.33784990929195,0.698756936804364));
#9567=CARTESIAN_POINT('Ctrl Pts',(11.399999182603,-1.33275899381189,0.699575346749464));
#9568=CARTESIAN_POINT('Ctrl Pts',(11.4000000015384,-1.32760128986121,0.699999998642559));
#9569=CARTESIAN_POINT('Ctrl Pts',(11.3999999999682,-1.32241589773435,0.7));
#9570=CARTESIAN_POINT('Ctrl Pts',(11.227882892666,-1.47337141465794,-0.000640335460849732));
#9571=CARTESIAN_POINT('Ctrl Pts',(11.218588765022,-1.46278323638644,0.201451598614313));
#9572=CARTESIAN_POINT('Ctrl Pts',(11.2092944683555,-1.45219508216535,0.40354352620373));
#9573=CARTESIAN_POINT('Ctrl Pts',(11.2000000000001,-1.44160695250309,0.60563544721184));
#9574=CARTESIAN_POINT('Ctrl Pts',(10.1843397214697,-1.57034855377304,-0.000384310983874139));
#9575=CARTESIAN_POINT('Ctrl Pts',(10.1768953195658,-1.55975965902304,0.201708049868595));
#9576=CARTESIAN_POINT('Ctrl Pts',(10.1694507716805,-1.54917076711515,0.403800406245857));
#9577=CARTESIAN_POINT('Ctrl Pts',(10.1620060668616,-1.53858190981164,0.605892758286982));
#9578=CARTESIAN_POINT('Ctrl Pts',(9.14170648965309,-1.65016851777514,-0.000148134864058495));
#9579=CARTESIAN_POINT('Ctrl Pts',(9.13611341817177,-1.63957870617509,0.201944615677573));
#9580=CARTESIAN_POINT('Ctrl Pts',(9.13052023035058,-1.6289888900612,0.404037363603497));
#9581=CARTESIAN_POINT('Ctrl Pts',(9.124926910836,-1.6183991014662,0.606130109186173));
#9582=CARTESIAN_POINT('Ctrl Pts',(8.1,-1.69866351109718,1.00613961606655E-16));
#9583=CARTESIAN_POINT('Ctrl Pts',(8.09625995443094,-1.68807302815665,0.202092993803311));
#9584=CARTESIAN_POINT('Ctrl Pts',(8.09251982249141,-1.67748255132318,0.404185986335255));
#9585=CARTESIAN_POINT('Ctrl Pts',(8.08877960280056,-1.66689208072706,0.606278977577217));
#9586=CARTESIAN_POINT('Ctrl Pts',(8.1,-1.66641703131627,0.605314487869832));
#9587=CARTESIAN_POINT('Ctrl Pts',(9.13548525483003,-1.617718421277,0.605389190939432));
#9588=CARTESIAN_POINT('Ctrl Pts',(10.168822041161,-1.53796707615457,0.605507632815633));
#9589=CARTESIAN_POINT('Ctrl Pts',(11.2000000000893,-1.44160695345912,0.605635447210802));
#9590=CARTESIAN_POINT('Ctrl Pts',(11.7095939787209,-1.42740645209206,-7.69249563980189E-5));
#9591=CARTESIAN_POINT('Ctrl Pts',(11.6994545874061,-1.41682738380082,0.201847033339061));
#9592=CARTESIAN_POINT('Ctrl Pts',(11.6893150192885,-1.40624834198077,0.403770984173611));
#9593=CARTESIAN_POINT('Ctrl Pts',(11.6791752715866,-1.39566932719028,0.605694927437301));
#9594=CARTESIAN_POINT('Ctrl Pts',(11.6063871276792,-1.43748358609578,-5.11721697277706E-5));
#9595=CARTESIAN_POINT('Ctrl Pts',(11.596430427176,-1.42690445239132,0.201872829148883));
#9596=CARTESIAN_POINT('Ctrl Pts',(11.5864735514701,-1.41632534465399,0.403796823219986));
#9597=CARTESIAN_POINT('Ctrl Pts',(11.5765164978042,-1.40574626343445,0.605720809936841));
#9598=CARTESIAN_POINT('Ctrl Pts',(11.5031891278894,-1.4474144288224,-2.55082377288765E-5));
#9599=CARTESIAN_POINT('Ctrl Pts',(11.4934151336386,-1.43683522760458,0.201898535909597));
#9600=CARTESIAN_POINT('Ctrl Pts',(11.4836409658656,-1.42625605183456,0.40382257302165));
#9601=CARTESIAN_POINT('Ctrl Pts',(11.4738666218385,-1.41567690205216,0.605746602994839));
#9602=CARTESIAN_POINT('Ctrl Pts',(11.4,-1.45718524058191,-5.20417042793042E-18));
#9603=CARTESIAN_POINT('Ctrl Pts',(11.3904087275488,-1.44660597001679,0.201924086674796));
#9604=CARTESIAN_POINT('Ctrl Pts',(11.3808172833376,-1.43602672436683,0.403848166524883));
#9605=CARTESIAN_POINT('Ctrl Pts',(11.3712256646606,-1.42544750415802,0.605772239449758));
#9606=CARTESIAN_POINT('',(11.6778970386953,-1.39579479040469,0.605695249702977));
#9607=CARTESIAN_POINT('Ctrl Pts',(11.4,-1.4227102204299,0.605660349289938));
#9608=CARTESIAN_POINT('Ctrl Pts',(11.4926474653491,-1.41386220753305,0.605671932550561));
#9609=CARTESIAN_POINT('Ctrl Pts',(11.585279512325,-1.40488700096013,0.605683574233495));
#9610=CARTESIAN_POINT('Ctrl Pts',(11.6778970386953,-1.39579479040469,0.605695249702977));
#9611=CARTESIAN_POINT('Ctrl Pts',(11.6778970386953,-1.39579479040469,0.605695249702977));
#9612=CARTESIAN_POINT('Ctrl Pts',(11.6884613130147,-1.40633044792991,0.403796817797553));
#9613=CARTESIAN_POINT('Ctrl Pts',(11.6990256725537,-1.41686632615463,0.201898401304098));
#9614=CARTESIAN_POINT('Ctrl Pts',(11.7095901160181,-1.42740242188993,5.19332840620557E-17));
#9615=CARTESIAN_POINT('Ctrl Pts',(11.2,-1.34133050917871,0.7));
#9616=CARTESIAN_POINT('Ctrl Pts',(10.1668086441106,-1.43797263608903,0.7));
#9617=CARTESIAN_POINT('Ctrl Pts',(9.13190264019122,-1.51792184128158,0.7));
#9618=CARTESIAN_POINT('Ctrl Pts',(8.09530923905977,-1.56666858280461,0.7));
#9619=CARTESIAN_POINT('Ctrl Pts',(11.2026864299662,-1.37005086445236,0.7));
#9620=CARTESIAN_POINT('Ctrl Pts',(10.1691860218014,-1.46674693471719,0.700000910790016));
#9621=CARTESIAN_POINT('Ctrl Pts',(9.13384227773975,-1.54675516497,0.699999464833944));
#9622=CARTESIAN_POINT('Ctrl Pts',(8.09666712422266,-1.59554384206015,0.700000000000001));
#9623=CARTESIAN_POINT('Ctrl Pts',(11.2073428085028,-1.4198317437391,0.676744232988519));
#9624=CARTESIAN_POINT('Ctrl Pts',(10.1733099382853,-1.51661799675652,0.676702307311825));
#9625=CARTESIAN_POINT('Ctrl Pts',(9.13719745543551,-1.59672983278297,0.676663906627884));
#9626=CARTESIAN_POINT('Ctrl Pts',(8.09902054834098,-1.64558911349573,0.676639354455264));
#9627=CARTESIAN_POINT('Ctrl Pts',(11.2091847227485,-1.43952346553595,0.627236497176141));
#9628=CARTESIAN_POINT('Ctrl Pts',(10.1749352046592,-1.53629892039422,0.62712791425818));
#9629=CARTESIAN_POINT('Ctrl Pts',(9.13852107143019,-1.61640633519008,0.627027713743691));
#9630=CARTESIAN_POINT('Ctrl Pts',(8.0999458765183,-1.66526610220338,0.626964226563296));
#9631=CARTESIAN_POINT('Ctrl Pts',(11.209298290232,-1.4407376041935,0.605636599993194));
#9632=CARTESIAN_POINT('Ctrl Pts',(10.1750338985877,-1.53748737250229,0.605508345221004));
#9633=CARTESIAN_POINT('Ctrl Pts',(9.13859765097935,-1.61757204607208,0.605389415477198));
#9634=CARTESIAN_POINT('Ctrl Pts',(8.1,-1.66641703131627,0.605314487869832));
#9635=CARTESIAN_POINT('Ctrl Pts',(11.2,-1.34133050917871,0.7));
#9636=CARTESIAN_POINT('Ctrl Pts',(10.16836710286,-1.43782686176815,0.7));
#9637=CARTESIAN_POINT('Ctrl Pts',(9.13502472651537,-1.51768061363633,0.7));
#9638=CARTESIAN_POINT('Ctrl Pts',(8.09999999865516,-1.56644778212326,0.7));
#9639=CARTESIAN_POINT('Ctrl Pts',(11.6681436286308,-1.2964346619681,0.7));
#9640=CARTESIAN_POINT('Ctrl Pts',(11.5756099286391,-1.3055179747114,0.7));
#9641=CARTESIAN_POINT('Ctrl Pts',(11.4830653488871,-1.31448403714215,0.7));
#9642=CARTESIAN_POINT('Ctrl Pts',(11.3905090053564,-1.32332268868375,0.7));
#9643=CARTESIAN_POINT('Ctrl Pts',(11.6709605510772,-1.32513126902304,0.700000000000001));
#9644=CARTESIAN_POINT('Ctrl Pts',(11.5784027531871,-1.33421922733773,0.700000082825348));
#9645=CARTESIAN_POINT('Ctrl Pts',(11.4858332859074,-1.34318985044544,0.699999917777441));
#9646=CARTESIAN_POINT('Ctrl Pts',(11.3932507170007,-1.35203326785046,0.7));
#9647=CARTESIAN_POINT('Ctrl Pts',(11.6758431636759,-1.37487151491717,0.67676311428296));
#9648=CARTESIAN_POINT('Ctrl Pts',(11.583243842395,-1.38396722707511,0.676759299309384));
#9649=CARTESIAN_POINT('Ctrl Pts',(11.4906306781253,-1.39294591144353,0.676755553516685));
#9650=CARTESIAN_POINT('Ctrl Pts',(11.3980029235659,-1.40179729139028,0.67675176769038));
#9651=CARTESIAN_POINT('Ctrl Pts',(11.6777767156198,-1.39456903283364,0.627286048421068));
#9652=CARTESIAN_POINT('Ctrl Pts',(11.5851604051362,-1.40366358810601,0.627276165220861));
#9653=CARTESIAN_POINT('Ctrl Pts',(11.4925297866457,-1.41264104586547,0.627266369072496));
#9654=CARTESIAN_POINT('Ctrl Pts',(11.3998836071583,-1.4214913811319,0.627256563056779));
#9655=CARTESIAN_POINT('Ctrl Pts',(11.6778970386953,-1.39579479040469,0.605695249702977));
#9656=CARTESIAN_POINT('Ctrl Pts',(11.585279512325,-1.40488700096013,0.605683574233495));
#9657=CARTESIAN_POINT('Ctrl Pts',(11.4926474653491,-1.41386220753305,0.605671932550561));
#9658=CARTESIAN_POINT('Ctrl Pts',(11.4,-1.4227102204299,0.605660349289938));
#9659=CARTESIAN_POINT('',(11.6681436286308,-1.2964346619681,0.7));
#9660=CARTESIAN_POINT('Ctrl Pts',(11.6681436286308,-1.2964346619681,0.7));
#9661=CARTESIAN_POINT('Ctrl Pts',(11.5787728332608,-1.30520749699507,0.7));
#9662=CARTESIAN_POINT('Ctrl Pts',(11.4893918891838,-1.31387096021207,0.7));
#9663=CARTESIAN_POINT('Ctrl Pts',(11.3999999999682,-1.32241589773435,0.7));
#9664=CARTESIAN_POINT('Origin',(11.6681436286308,-1.2964346619681,0.6));
#9665=CARTESIAN_POINT('Origin',(6.08012166120517,1.06778195214465E-16,0.7));
#9666=CARTESIAN_POINT('Ctrl Pts',(8.0999999986552,1.56644778212326,0.7));
#9667=CARTESIAN_POINT('Ctrl Pts',(9.13502472651542,1.51768061363633,0.7));
#9668=CARTESIAN_POINT('Ctrl Pts',(10.16836710286,1.43782686176815,0.7));
#9669=CARTESIAN_POINT('Ctrl Pts',(11.2,1.34133050917871,0.7));
#9670=CARTESIAN_POINT('Origin',(6.08012166120517,1.06778195214465E-16,0.7));
#9671=CARTESIAN_POINT('',(11.6681436286308,1.2964346619681,0.7));
#9672=CARTESIAN_POINT('Ctrl Pts',(11.3999999999682,1.32241589773435,0.7));
#9673=CARTESIAN_POINT('Ctrl Pts',(11.4893918891837,1.31387096021208,0.7));
#9674=CARTESIAN_POINT('Ctrl Pts',(11.5787728332608,1.30520749699508,0.7));
#9675=CARTESIAN_POINT('Ctrl Pts',(11.6681436286308,1.2964346619681,0.7));
#9676=CARTESIAN_POINT('',(11.6681436286308,0.8,0.7));
#9677=CARTESIAN_POINT('Ctrl Pts',(8.09530923905978,1.56666858280461,0.7));
#9678=CARTESIAN_POINT('Ctrl Pts',(9.13190264019124,1.51792184128158,0.7));
#9679=CARTESIAN_POINT('Ctrl Pts',(10.1668086441106,1.43797263608903,0.7));
#9680=CARTESIAN_POINT('Ctrl Pts',(11.2,1.34133050917871,0.7));
#9681=CARTESIAN_POINT('Ctrl Pts',(8.09666712422266,1.59554384206015,0.700000000000001));
#9682=CARTESIAN_POINT('Ctrl Pts',(9.13384227773977,1.54675516497,0.699999464833944));
#9683=CARTESIAN_POINT('Ctrl Pts',(10.1691860218013,1.46674693471719,0.700000910790016));
#9684=CARTESIAN_POINT('Ctrl Pts',(11.2026864299662,1.37005086445236,0.7));
#9685=CARTESIAN_POINT('Ctrl Pts',(8.09902054834099,1.64558911349573,0.676639354455264));
#9686=CARTESIAN_POINT('Ctrl Pts',(9.13719745543553,1.59672983278297,0.676663906627884));
#9687=CARTESIAN_POINT('Ctrl Pts',(10.1733099382853,1.51661799675652,0.676702307311825));
#9688=CARTESIAN_POINT('Ctrl Pts',(11.2073428085028,1.4198317437391,0.676744232988519));
#9689=CARTESIAN_POINT('Ctrl Pts',(8.0999458765183,1.66526610220338,0.626964226563296));
#9690=CARTESIAN_POINT('Ctrl Pts',(9.1385210714302,1.61640633519008,0.627027713743691));
#9691=CARTESIAN_POINT('Ctrl Pts',(10.1749352046592,1.53629892039423,0.62712791425818));
#9692=CARTESIAN_POINT('Ctrl Pts',(11.2091847227485,1.43952346553595,0.627236497176141));
#9693=CARTESIAN_POINT('Ctrl Pts',(8.1,1.66641703131627,0.605314487869832));
#9694=CARTESIAN_POINT('Ctrl Pts',(9.13859765097937,1.61757204607208,0.605389415477198));
#9695=CARTESIAN_POINT('Ctrl Pts',(10.1750338985877,1.53748737250229,0.605508345221004));
#9696=CARTESIAN_POINT('Ctrl Pts',(11.209298290232,1.4407376041935,0.605636599993194));
#9697=CARTESIAN_POINT('Ctrl Pts',(11.2000000000893,1.44160695345912,0.605635447210802));
#9698=CARTESIAN_POINT('Ctrl Pts',(10.168822041161,1.53796707615457,0.605507632815633));
#9699=CARTESIAN_POINT('Ctrl Pts',(9.13548525483005,1.617718421277,0.605389190939432));
#9700=CARTESIAN_POINT('Ctrl Pts',(8.1,1.66641703131627,0.605314487869832));
#9701=CARTESIAN_POINT('Ctrl Pts',(8.1,1.69866351109859,-2.6441702993818E-11));
#9702=CARTESIAN_POINT('Ctrl Pts',(8.09625995443078,1.68807302815759,0.202092993785684));
#9703=CARTESIAN_POINT('Ctrl Pts',(8.09251982249108,1.67748255132366,0.404185986326441));
#9704=CARTESIAN_POINT('Ctrl Pts',(8.08877960280008,1.66689208072708,0.606278977577217));
#9705=CARTESIAN_POINT('Ctrl Pts',(9.14170648965349,1.65016851777655,-0.00014813489050026));
#9706=CARTESIAN_POINT('Ctrl Pts',(9.13611341817193,1.63957870617604,0.201944615659945));
#9707=CARTESIAN_POINT('Ctrl Pts',(9.1305202303505,1.62898889006169,0.404037363594684));
#9708=CARTESIAN_POINT('Ctrl Pts',(9.12492691083567,1.61839910146622,0.606130109186173));
#9709=CARTESIAN_POINT('Ctrl Pts',(10.1843397214705,1.57034855377444,-0.000384311010315772));
#9710=CARTESIAN_POINT('Ctrl Pts',(10.1768953195662,1.55975965902398,0.201708049850968));
#9711=CARTESIAN_POINT('Ctrl Pts',(10.1694507716807,1.54917076711562,0.403800406237042));
#9712=CARTESIAN_POINT('Ctrl Pts',(10.1620060668615,1.53858190981166,0.605892758286982));
#9713=CARTESIAN_POINT('Ctrl Pts',(11.2278828926672,1.47337141465933,-0.000640335487291374));
#9714=CARTESIAN_POINT('Ctrl Pts',(11.2185887650228,1.46278323638736,0.201451598596686));
#9715=CARTESIAN_POINT('Ctrl Pts',(11.2092944683559,1.45219508216582,0.403543526194916));
#9716=CARTESIAN_POINT('Ctrl Pts',(11.2000000000001,1.44160695250309,0.60563544721184));
#9717=CARTESIAN_POINT('Ctrl Pts',(11.4,1.45718524058191,-1.37043154602168E-16));
#9718=CARTESIAN_POINT('Ctrl Pts',(11.3904087275488,1.44660597001679,0.201924086674796));
#9719=CARTESIAN_POINT('Ctrl Pts',(11.3808172833376,1.43602672436683,0.403848166524884));
#9720=CARTESIAN_POINT('Ctrl Pts',(11.3712256646606,1.42544750415802,0.605772239449759));
#9721=CARTESIAN_POINT('Ctrl Pts',(11.5031891278894,1.4474144288224,-2.55082377290153E-5));
#9722=CARTESIAN_POINT('Ctrl Pts',(11.4934151336386,1.43683522760458,0.201898535909598));
#9723=CARTESIAN_POINT('Ctrl Pts',(11.4836409658656,1.42625605183455,0.40382257302165));
#9724=CARTESIAN_POINT('Ctrl Pts',(11.4738666218385,1.41567690205216,0.605746602994839));
#9725=CARTESIAN_POINT('Ctrl Pts',(11.6063871276792,1.43748358609579,-5.1172169727805E-5));
#9726=CARTESIAN_POINT('Ctrl Pts',(11.596430427176,1.42690445239132,0.201872829148883));
#9727=CARTESIAN_POINT('Ctrl Pts',(11.5864735514701,1.41632534465399,0.403796823219986));
#9728=CARTESIAN_POINT('Ctrl Pts',(11.5765164978042,1.40574626343445,0.605720809936842));
#9729=CARTESIAN_POINT('Ctrl Pts',(11.7095939787209,1.42740645209206,-7.69249563980588E-5));
#9730=CARTESIAN_POINT('Ctrl Pts',(11.6994545874061,1.41682738380082,0.201847033339061));
#9731=CARTESIAN_POINT('Ctrl Pts',(11.6893150192885,1.40624834198077,0.403770984173611));
#9732=CARTESIAN_POINT('Ctrl Pts',(11.6791752715866,1.39566932719028,0.605694927437301));
#9733=CARTESIAN_POINT('',(11.6778970386953,1.39579479040469,0.605695249702977));
#9734=CARTESIAN_POINT('Ctrl Pts',(11.7095901160181,1.42740242188993,2.01986864734049E-16));
#9735=CARTESIAN_POINT('Ctrl Pts',(11.6990256725537,1.41686632615463,0.201898401304098));
#9736=CARTESIAN_POINT('Ctrl Pts',(11.6884613130147,1.40633044792991,0.403796817797553));
#9737=CARTESIAN_POINT('Ctrl Pts',(11.6778970386953,1.39579479040469,0.605695249702978));
#9738=CARTESIAN_POINT('Ctrl Pts',(11.6778970386953,1.39579479040469,0.605695249702977));
#9739=CARTESIAN_POINT('Ctrl Pts',(11.585279512325,1.40488700096013,0.605683574233495));
#9740=CARTESIAN_POINT('Ctrl Pts',(11.4926474653491,1.41386220753305,0.605671932550561));
#9741=CARTESIAN_POINT('Ctrl Pts',(11.4,1.4227102204299,0.605660349289938));
#9742=CARTESIAN_POINT('Origin',(7.9,1.7737037037037,0.));
#9743=CARTESIAN_POINT('',(7.9,-1.67543132363858,0.605300614462415));
#9744=CARTESIAN_POINT('Ctrl Pts',(7.9,-1.67543132363858,0.605300614462415));
#9745=CARTESIAN_POINT('Ctrl Pts',(7.9,-1.68078196203297,0.504592238472094));
#9746=CARTESIAN_POINT('Ctrl Pts',(7.9,-1.68613236521525,0.403883028813119));
#9747=CARTESIAN_POINT('Ctrl Pts',(7.9,-1.69685110017509,0.202116711316755));
#9748=CARTESIAN_POINT('Ctrl Pts',(7.9,-1.70221951791351,0.10105794916591));
#9749=CARTESIAN_POINT('Ctrl Pts',(7.9,-1.70758761671949,0.));
#9750=CARTESIAN_POINT('',(7.9,-1.57547905376932,0.7));
#9751=CARTESIAN_POINT('Ctrl Pts',(7.9,-1.57547905376882,0.7));
#9752=CARTESIAN_POINT('Ctrl Pts',(7.9,-1.58339333479856,0.700000000000001));
#9753=CARTESIAN_POINT('Ctrl Pts',(7.89999913038498,-1.59124411312484,0.699006032637452));
#9754=CARTESIAN_POINT('Ctrl Pts',(7.89999837104309,-1.59889106951376,0.697118831203047));
#9755=CARTESIAN_POINT('Ctrl Pts',(7.89999794343345,-1.6031973145812,0.696056087876834));
#9756=CARTESIAN_POINT('Ctrl Pts',(7.89999755365678,-1.60743898057435,0.694709047589066));
#9757=CARTESIAN_POINT('Ctrl Pts',(7.89999730661842,-1.61158931211603,0.693088720937666));
#9758=CARTESIAN_POINT('Ctrl Pts',(7.89999686465941,-1.6190143793929,0.690189908089508));
#9759=CARTESIAN_POINT('Ctrl Pts',(7.89999696143539,-1.626066934352,0.686450944759811));
#9760=CARTESIAN_POINT('Ctrl Pts',(7.89999752554231,-1.63260082031789,0.681953255064161));
#9761=CARTESIAN_POINT('Ctrl Pts',(7.89999783650325,-1.63620259020663,0.679473927540052));
#9762=CARTESIAN_POINT('Ctrl Pts',(7.89999827825103,-1.63964648551863,0.676763160200805));
#9763=CARTESIAN_POINT('Ctrl Pts',(7.89999867021687,-1.64290407802379,0.673829034208746));
#9764=CARTESIAN_POINT('Ctrl Pts',(7.89999905115172,-1.64606999298761,0.670977482527793));
#9765=CARTESIAN_POINT('Ctrl Pts',(7.89999938859403,-1.64904076201529,0.667932171841817));
#9766=CARTESIAN_POINT('Ctrl Pts',(7.89999938783828,-1.6517939440564,0.66470449824639));
#9767=CARTESIAN_POINT('Ctrl Pts',(7.89999938643498,-1.65690611124346,0.658711285012161));
#9768=CARTESIAN_POINT('Ctrl Pts',(7.89999834643869,-1.661271022418,0.652090721578155));
#9769=CARTESIAN_POINT('Ctrl Pts',(7.89999799057748,-1.66482884904143,0.645008203309728));
#9770=CARTESIAN_POINT('Ctrl Pts',(7.89999795399159,-1.66519462718329,0.644280053614395));
#9771=CARTESIAN_POINT('Ctrl Pts',(7.89999792287445,-1.66555183396469,0.643547001244109));
#9772=CARTESIAN_POINT('Ctrl Pts',(7.89999789784292,-1.66590037542058,0.642809214685104));
#9773=CARTESIAN_POINT('Ctrl Pts',(7.89999765441981,-1.66928982250308,0.635634491398386));
#9774=CARTESIAN_POINT('Ctrl Pts',(7.89999817709027,-1.67182454272713,0.628096763436417));
#9775=CARTESIAN_POINT('Ctrl Pts',(7.8999989464625,-1.67345106343068,0.620364350320046));
#9776=CARTESIAN_POINT('Ctrl Pts',(7.89999943944948,-1.67449328136075,0.615409688768565));
#9777=CARTESIAN_POINT('Ctrl Pts',(7.89999999630063,-1.67516175160204,0.610374426093907));
#9778=CARTESIAN_POINT('Ctrl Pts',(7.89999999769359,-1.67543132314592,0.605300614465834));
#9779=CARTESIAN_POINT('',(7.9,1.57547905376882,0.7));
#9780=CARTESIAN_POINT('',(7.9,0.886851851851852,0.7));
#9781=CARTESIAN_POINT('',(7.9,1.67543132363858,0.605300614462415));
#9782=CARTESIAN_POINT('Ctrl Pts',(7.89999999769359,1.67543132314592,0.605300614465834));
#9783=CARTESIAN_POINT('Ctrl Pts',(7.89999999552123,1.67501091691767,0.613213400729193));
#9784=CARTESIAN_POINT('Ctrl Pts',(7.89999875799714,1.67362284400845,0.621034919585595));
#9785=CARTESIAN_POINT('Ctrl Pts',(7.89999821041927,1.67135120200026,0.628604813990272));
#9786=CARTESIAN_POINT('Ctrl Pts',(7.89999790518813,1.67008494211401,0.632824428521627));
#9787=CARTESIAN_POINT('Ctrl Pts',(7.89999777089825,1.66854314417455,0.636965893954691));
#9788=CARTESIAN_POINT('Ctrl Pts',(7.89999784944871,1.66673368022774,0.640999456224326));
#9789=CARTESIAN_POINT('Ctrl Pts',(7.89999799035603,1.66348778281681,0.648235040746992));
#9790=CARTESIAN_POINT('Ctrl Pts',(7.8999989183875,1.65941887886545,0.655045206964536));
#9791=CARTESIAN_POINT('Ctrl Pts',(7.89999927807636,1.65459101651367,0.661266862646797));
#9792=CARTESIAN_POINT('Ctrl Pts',(7.89999934554656,1.65368540929837,0.662433916689859));
#9793=CARTESIAN_POINT('Ctrl Pts',(7.89999938740919,1.65275296801062,0.663580193269421));
#9794=CARTESIAN_POINT('Ctrl Pts',(7.89999938728957,1.65179394408007,0.664704498246374));
#9795=CARTESIAN_POINT('Ctrl Pts',(7.89999938705343,1.64990069294102,0.666924037937161));
#9796=CARTESIAN_POINT('Ctrl Pts',(7.89999922461202,1.64790387543569,0.669057997255949));
#9797=CARTESIAN_POINT('Ctrl Pts',(7.89999900301747,1.64581073954063,0.671102663899023));
#9798=CARTESIAN_POINT('Ctrl Pts',(7.89999840121276,1.64012621790684,0.676655553128015));
#9799=CARTESIAN_POINT('Ctrl Pts',(7.89999746538644,1.63379824275617,0.681490110487894));
#9800=CARTESIAN_POINT('Ctrl Pts',(7.89999715581736,1.6269906793715,0.685552192443336));
#9801=CARTESIAN_POINT('Ctrl Pts',(7.89999695885968,1.62265949106942,0.688136618155352));
#9802=CARTESIAN_POINT('Ctrl Pts',(7.89999697413705,1.61813320929371,0.690407672840119));
#9803=CARTESIAN_POINT('Ctrl Pts',(7.89999720528031,1.61344832872307,0.692342105328139));
#9804=CARTESIAN_POINT('Ctrl Pts',(7.89999756646959,1.60612763680413,0.69536488980882));
#9805=CARTESIAN_POINT('Ctrl Pts',(7.89999845750109,1.59850458633822,0.69753330980446));
#9806=CARTESIAN_POINT('Ctrl Pts',(7.89999917312139,1.59072625322659,0.698777780766876));
#9807=CARTESIAN_POINT('Ctrl Pts',(7.8999996358458,1.58569673594883,0.699582463224842));
#9808=CARTESIAN_POINT('Ctrl Pts',(7.9,1.58060170040825,0.7));
#9809=CARTESIAN_POINT('Ctrl Pts',(7.9,1.57547905376882,0.7));
#9810=CARTESIAN_POINT('Ctrl Pts',(7.9,1.70758761671949,0.));
#9811=CARTESIAN_POINT('Ctrl Pts',(7.9,1.70221949782947,0.101058327261027));
#9812=CARTESIAN_POINT('Ctrl Pts',(7.9,1.69685105999395,0.202117467714));
#9813=CARTESIAN_POINT('Ctrl Pts',(7.9,1.68613232500772,0.403883785628764));
#9814=CARTESIAN_POINT('Ctrl Pts',(7.9,1.6807819419292,0.504592616860323));
#9815=CARTESIAN_POINT('Ctrl Pts',(7.9,1.67543132363858,0.605300614462415));
#9816=CARTESIAN_POINT('Ctrl Pts',(7.91019312999368,-1.70715886092982,-0.000134090250286965));
#9817=CARTESIAN_POINT('Ctrl Pts',(7.90679525219671,-1.69658223918655,0.201692187253877));
#9818=CARTESIAN_POINT('Ctrl Pts',(7.90339729501941,-1.68600562260833,0.40351846369823));
#9819=CARTESIAN_POINT('Ctrl Pts',(7.89999925719352,-1.67542901130525,0.605344739067286));
#9820=CARTESIAN_POINT('Ctrl Pts',(6.63535348802246,-1.76179300886274,3.38453142643293E-5));
#9821=CARTESIAN_POINT('Ctrl Pts',(6.63422081661327,-1.7512156246026,0.201860399405878));
#9822=CARTESIAN_POINT('Ctrl Pts',(6.6330881724013,-1.74063821514668,0.403686949685767));
#9823=CARTESIAN_POINT('Ctrl Pts',(6.63195543348167,-1.7300608292057,0.605513504373875));
#9824=CARTESIAN_POINT('Ctrl Pts',(5.36191629096386,-1.76821426310706,6.25694230841134E-5));
#9825=CARTESIAN_POINT('Ctrl Pts',(5.36305144950513,-1.75763653444312,0.201889164820622));
#9826=CARTESIAN_POINT('Ctrl Pts',(5.36418670601529,-1.74705878452761,0.403715755186214));
#9827=CARTESIAN_POINT('Ctrl Pts',(5.36532191986746,-1.73648104871457,0.605542351516859));
#9828=CARTESIAN_POINT('Ctrl Pts',(4.08978435919194,-1.70060618495018,-0.000163379468877527));
#9829=CARTESIAN_POINT('Ctrl Pts',(4.09318947412453,-1.69002991101751,0.201662855819258));
#9830=CARTESIAN_POINT('Ctrl Pts',(4.09659468720556,-1.67945364498778,0.403489089874722));
#9831=CARTESIAN_POINT('Ctrl Pts',(4.1,-1.66887738702936,0.605315322680078));
#9832=CARTESIAN_POINT('Ctrl Pts',(4.10000000006189,-1.66887738587128,0.605315322687833));
#9833=CARTESIAN_POINT('Ctrl Pts',(5.36600428635239,-1.73653511802878,0.605201749988751));
#9834=CARTESIAN_POINT('Ctrl Pts',(6.63469107356441,-1.72995836404769,0.605216415547347));
#9835=CARTESIAN_POINT('Ctrl Pts',(7.89999999997453,-1.67543132304763,0.605300614465986));
#9836=CARTESIAN_POINT('Ctrl Pts',(7.9,-1.57547905376882,0.7));
#9837=CARTESIAN_POINT('Ctrl Pts',(6.63400208894818,-1.63014048526579,0.7));
#9838=CARTESIAN_POINT('Ctrl Pts',(5.36531976402288,-1.63670020240541,0.7));
#9839=CARTESIAN_POINT('Ctrl Pts',(4.09999999999999,-1.56887583540973,0.7));
#9840=CARTESIAN_POINT('Ctrl Pts',(7.9012470621039,-1.60436190544783,0.700000000000001));
#9841=CARTESIAN_POINT('Ctrl Pts',(6.6345175325877,-1.65907137725265,0.700000604190856));
#9842=CARTESIAN_POINT('Ctrl Pts',(5.36490325870521,-1.66564852467601,0.700000815814724));
#9843=CARTESIAN_POINT('Ctrl Pts',(4.09845273665223,-1.59774131518914,0.699999999999999));
#9844=CARTESIAN_POINT('Ctrl Pts',(7.90340849276168,-1.6544221878571,0.676636720659303));
#9845=CARTESIAN_POINT('Ctrl Pts',(6.63541917043928,-1.70921256696412,0.676609005714152));
#9846=CARTESIAN_POINT('Ctrl Pts',(5.36416860778507,-1.71581908642683,0.67660414986632));
#9847=CARTESIAN_POINT('Ctrl Pts',(4.09577098158984,-1.64777167791894,0.676641578059328));
#9848=CARTESIAN_POINT('Ctrl Pts',(7.90425799286387,-1.67409721877663,0.626952737571144));
#9849=CARTESIAN_POINT('Ctrl Pts',(6.63576820027036,-1.72888861107585,0.626881076846221));
#9850=CARTESIAN_POINT('Ctrl Pts',(5.36388821219926,-1.73550154452763,0.626868555890157));
#9851=CARTESIAN_POINT('Ctrl Pts',(4.09471668402893,-1.66744047248441,0.626965338598652));
#9852=CARTESIAN_POINT('Ctrl Pts',(7.90430757201307,-1.67524550738887,0.605300901379154));
#9853=CARTESIAN_POINT('Ctrl Pts',(6.63578978311492,-1.73002023206136,0.605216330280387));
#9854=CARTESIAN_POINT('Ctrl Pts',(5.3638700255334,-1.7366305488338,0.605201579557148));
#9855=CARTESIAN_POINT('Ctrl Pts',(4.09465499692593,-1.6685912965035,0.605315802949303));
#9856=CARTESIAN_POINT('Ctrl Pts',(7.9,-1.57547905376882,0.7));
#9857=CARTESIAN_POINT('Ctrl Pts',(6.63400208894818,-1.63014048526579,0.7));
#9858=CARTESIAN_POINT('Ctrl Pts',(5.36531976402288,-1.63670020240541,0.7));
#9859=CARTESIAN_POINT('Ctrl Pts',(4.09999999999999,-1.56887583540973,0.7));
#9860=CARTESIAN_POINT('Origin',(6.08012166120517,1.06778195214465E-16,0.7));
#9861=CARTESIAN_POINT('Ctrl Pts',(4.1,1.56887583540973,0.7));
#9862=CARTESIAN_POINT('Ctrl Pts',(5.36531976402291,1.63670020240541,0.7));
#9863=CARTESIAN_POINT('Ctrl Pts',(6.63400208894819,1.63014048526579,0.7));
#9864=CARTESIAN_POINT('Ctrl Pts',(7.9,1.57547905376882,0.7));
#9865=CARTESIAN_POINT('Ctrl Pts',(4.1,1.56887583540973,0.7));
#9866=CARTESIAN_POINT('Ctrl Pts',(5.36531976402291,1.63670020240541,0.7));
#9867=CARTESIAN_POINT('Ctrl Pts',(6.63400208894819,1.63014048526579,0.7));
#9868=CARTESIAN_POINT('Ctrl Pts',(7.9,1.57547905376882,0.7));
#9869=CARTESIAN_POINT('Ctrl Pts',(4.09845273665224,1.59774131518914,0.699999999999999));
#9870=CARTESIAN_POINT('Ctrl Pts',(5.36490325870523,1.66564852467601,0.700000815814725));
#9871=CARTESIAN_POINT('Ctrl Pts',(6.6345175325877,1.65907137725265,0.700000604190856));
#9872=CARTESIAN_POINT('Ctrl Pts',(7.9012470621039,1.60436190544783,0.700000000000001));
#9873=CARTESIAN_POINT('Ctrl Pts',(4.09577098158985,1.64777167791894,0.676641578059328));
#9874=CARTESIAN_POINT('Ctrl Pts',(5.36416860778509,1.71581908642683,0.67660414986632));
#9875=CARTESIAN_POINT('Ctrl Pts',(6.6354191704393,1.70921256696412,0.676609005714152));
#9876=CARTESIAN_POINT('Ctrl Pts',(7.90340849276168,1.6544221878571,0.676636720659302));
#9877=CARTESIAN_POINT('Ctrl Pts',(4.09471668402895,1.66744047248441,0.626965338598652));
#9878=CARTESIAN_POINT('Ctrl Pts',(5.36388821219928,1.73550154452763,0.626868555890157));
#9879=CARTESIAN_POINT('Ctrl Pts',(6.63576820027036,1.72888861107585,0.626881076846221));
#9880=CARTESIAN_POINT('Ctrl Pts',(7.90425799286387,1.67409721877663,0.626952737571144));
#9881=CARTESIAN_POINT('Ctrl Pts',(4.09465499692594,1.6685912965035,0.605315802949303));
#9882=CARTESIAN_POINT('Ctrl Pts',(5.36387002553342,1.7366305488338,0.605201579557148));
#9883=CARTESIAN_POINT('Ctrl Pts',(6.63578978311492,1.73002023206136,0.605216330280387));
#9884=CARTESIAN_POINT('Ctrl Pts',(7.90430757201307,1.67524550738887,0.605300901379154));
#9885=CARTESIAN_POINT('Ctrl Pts',(7.89999999997454,1.67543132304763,0.605300614465986));
#9886=CARTESIAN_POINT('Ctrl Pts',(6.63469107356441,1.72995836404769,0.605216415547348));
#9887=CARTESIAN_POINT('Ctrl Pts',(5.36600428635241,1.73653511802878,0.605201749988751));
#9888=CARTESIAN_POINT('Ctrl Pts',(4.10000000006189,1.66887738587128,0.605315322687833));
#9889=CARTESIAN_POINT('Ctrl Pts',(4.08978435969213,1.70060618339657,-0.000163349821525811));
#9890=CARTESIAN_POINT('Ctrl Pts',(4.093189474458,1.69002990998177,0.201662875584159));
#9891=CARTESIAN_POINT('Ctrl Pts',(4.0965946873723,1.67945364446992,0.403489099757173));
#9892=CARTESIAN_POINT('Ctrl Pts',(4.1,1.66887738702936,0.605315322680078));
#9893=CARTESIAN_POINT('Ctrl Pts',(5.36191629113061,1.76821426155324,6.25990704884337E-5));
#9894=CARTESIAN_POINT('Ctrl Pts',(5.3630514496163,1.75763653340724,0.201889184585558));
#9895=CARTESIAN_POINT('Ctrl Pts',(5.36418670607087,1.74705878400967,0.403715765068683));
#9896=CARTESIAN_POINT('Ctrl Pts',(5.36532191986745,1.73648104871457,0.605542351516858));
#9897=CARTESIAN_POINT('Ctrl Pts',(6.63535348785608,1.76179300730897,3.38749616628245E-5));
#9898=CARTESIAN_POINT('Ctrl Pts',(6.63422081650235,1.75121562356675,0.20186041917081));
#9899=CARTESIAN_POINT('Ctrl Pts',(6.63308817234583,1.74063821462875,0.403686959568233));
#9900=CARTESIAN_POINT('Ctrl Pts',(6.63195543348166,1.7300608292057,0.605513504373875));
#9901=CARTESIAN_POINT('Ctrl Pts',(7.91019312949454,1.70715885937616,-0.000134060602928919));
#9902=CARTESIAN_POINT('Ctrl Pts',(7.90679525186394,1.69658223815078,0.201692207018782));
#9903=CARTESIAN_POINT('Ctrl Pts',(7.90339729485302,1.68600562209044,0.403518473580683));
#9904=CARTESIAN_POINT('Ctrl Pts',(7.89999925719352,1.67542901130525,0.605344739067286));
#9905=CARTESIAN_POINT('Origin',(3.9,1.7662962962963,0.));
#9906=CARTESIAN_POINT('',(3.9,-1.657567947596,0.605334330700044));
#9907=CARTESIAN_POINT('Ctrl Pts',(3.9,-1.657567947596,0.605334330700044));
#9908=CARTESIAN_POINT('Ctrl Pts',(3.9,-1.66295505583237,0.504667750148195));
#9909=CARTESIAN_POINT('Ctrl Pts',(3.9,-1.66834175427306,0.404000185805616));
#9910=CARTESIAN_POINT('Ctrl Pts',(3.9,-1.67913790341918,0.202222727053817));
#9911=CARTESIAN_POINT('Ctrl Pts',(3.9,-1.68454745406112,0.101110889248462));
#9912=CARTESIAN_POINT('Ctrl Pts',(3.9,-1.68995649764597,0.));
#9913=CARTESIAN_POINT('',(3.9,-1.55753217754889,0.7));
#9914=CARTESIAN_POINT('Ctrl Pts',(3.89999999700315,-1.55753217437,0.7));
#9915=CARTESIAN_POINT('Ctrl Pts',(3.89999999197785,-1.56545359401377,0.699999998841372));
#9916=CARTESIAN_POINT('Ctrl Pts',(3.90000117861029,-1.57331197233837,0.699006163267487));
#9917=CARTESIAN_POINT('Ctrl Pts',(3.90000221019459,-1.58096665047841,0.697118921400131));
#9918=CARTESIAN_POINT('Ctrl Pts',(3.90000279139136,-1.58527931230009,0.696055645348449));
#9919=CARTESIAN_POINT('Ctrl Pts',(3.90000331912093,-1.58952737074567,0.694707745526415));
#9920=CARTESIAN_POINT('Ctrl Pts',(3.90000364796674,-1.59368396010392,0.693086194530447));
#9921=CARTESIAN_POINT('Ctrl Pts',(3.90000423564848,-1.60111221870485,0.690188313817561));
#9922=CARTESIAN_POINT('Ctrl Pts',(3.90000407815102,-1.60816848972648,0.686450841450731));
#9923=CARTESIAN_POINT('Ctrl Pts',(3.9000032813392,-1.6147063365644,0.681954558458482));
#9924=CARTESIAN_POINT('Ctrl Pts',(3.90000284137901,-1.61831621321653,0.679471932695374));
#9925=CARTESIAN_POINT('Ctrl Pts',(3.90000222202081,-1.62176776859012,0.67675708350434));
#9926=CARTESIAN_POINT('Ctrl Pts',(3.9000016760669,-1.6250323621476,0.673818036286869));
#9927=CARTESIAN_POINT('Ctrl Pts',(3.90000114791654,-1.62819049732732,0.670974831382826));
#9928=CARTESIAN_POINT('Ctrl Pts',(3.90000068451114,-1.63115458712464,0.667938911589952));
#9929=CARTESIAN_POINT('Ctrl Pts',(3.90000068976928,-1.6339023205034,0.664721489040691));
#9930=CARTESIAN_POINT('Ctrl Pts',(3.90000069956116,-1.63901923218135,0.658729908073458));
#9931=CARTESIAN_POINT('Ctrl Pts',(3.9000021571807,-1.64338878348726,0.652110283780478));
#9932=CARTESIAN_POINT('Ctrl Pts',(3.90000267296827,-1.64695081636755,0.645027851744832));
#9933=CARTESIAN_POINT('Ctrl Pts',(3.90000272641596,-1.64731992654249,0.644293945625623));
#9934=CARTESIAN_POINT('Ctrl Pts',(3.90000277224081,-1.64768032438231,0.643555049900053));
#9935=CARTESIAN_POINT('Ctrl Pts',(3.90000280957334,-1.64803191324525,0.642811337026806));
#9936=CARTESIAN_POINT('Ctrl Pts',(3.90000316967295,-1.65142324611312,0.635637680016741));
#9937=CARTESIAN_POINT('Ctrl Pts',(3.90000247513984,-1.65395957542788,0.628100801230905));
#9938=CARTESIAN_POINT('Ctrl Pts',(3.90000142932204,-1.65558732484325,0.62036898832433));
#9939=CARTESIAN_POINT('Ctrl Pts',(3.90000076044003,-1.65662839749185,0.615423891207338));
#9940=CARTESIAN_POINT('Ctrl Pts',(3.9,-1.65729694754734,0.61039839235075));
#9941=CARTESIAN_POINT('Ctrl Pts',(3.9,-1.657567947596,0.605334330700044));
#9942=CARTESIAN_POINT('',(3.9,1.55753217754922,0.7));
#9943=CARTESIAN_POINT('',(3.9,0.883148148148148,0.7));
#9944=CARTESIAN_POINT('',(3.9,1.657567947596,0.605334330700044));
#9945=CARTESIAN_POINT('Ctrl Pts',(3.9,1.657567947596,0.605334330700044));
#9946=CARTESIAN_POINT('Ctrl Pts',(3.9,1.65714453107083,0.613246533660879));
#9947=CARTESIAN_POINT('Ctrl Pts',(3.90000169450566,1.65575314729854,0.621067109624563));
#9948=CARTESIAN_POINT('Ctrl Pts',(3.900002426785,1.653477907766,0.628635640467799));
#9949=CARTESIAN_POINT('Ctrl Pts',(3.90000283370343,1.65221358571927,0.632841378048222));
#9950=CARTESIAN_POINT('Ctrl Pts',(3.90000300372053,1.65067534627202,0.636969322077829));
#9951=CARTESIAN_POINT('Ctrl Pts',(3.90000288278183,1.6488710006323,0.640990000951852));
#9952=CARTESIAN_POINT('Ctrl Pts',(3.90000266510116,1.6456233127241,0.64822692378658));
#9953=CARTESIAN_POINT('Ctrl Pts',(3.90000136145047,1.64155197609259,0.655037842274187));
#9954=CARTESIAN_POINT('Ctrl Pts',(3.9000008487987,1.63672139510901,0.661259788874982));
#9955=CARTESIAN_POINT('Ctrl Pts',(3.90000075195303,1.63580884415802,0.662435184403355));
#9956=CARTESIAN_POINT('Ctrl Pts',(3.90000069125178,1.63486906637168,0.663589490553999));
#9957=CARTESIAN_POINT('Ctrl Pts',(3.90000068992127,1.63390232051248,0.664721489040685));
#9958=CARTESIAN_POINT('Ctrl Pts',(3.90000068733544,1.63202347103487,0.666921503393101));
#9959=CARTESIAN_POINT('Ctrl Pts',(3.9000009071255,1.6300427915863,0.669037305429552));
#9960=CARTESIAN_POINT('Ctrl Pts',(3.90000121037842,1.62796736695056,0.671065303566633));
#9961=CARTESIAN_POINT('Ctrl Pts',(3.90000204102081,1.62228255539437,0.676620208836154));
#9962=CARTESIAN_POINT('Ctrl Pts',(3.90000335328325,1.61595386407616,0.681456575151491));
#9963=CARTESIAN_POINT('Ctrl Pts',(3.90000380482706,1.60914557515952,0.685520902406533));
#9964=CARTESIAN_POINT('Ctrl Pts',(3.90000409284089,1.60480295930069,0.688113302965514));
#9965=CARTESIAN_POINT('Ctrl Pts',(3.90000408819389,1.6002642541482,0.690390927291682));
#9966=CARTESIAN_POINT('Ctrl Pts',(3.90000378365133,1.59556629223371,0.692330537597694));
#9967=CARTESIAN_POINT('Ctrl Pts',(3.90000330864444,1.58823869807682,0.695355823328757));
#9968=CARTESIAN_POINT('Ctrl Pts',(3.90000209726118,1.58060840086481,0.697526456028474));
#9969=CARTESIAN_POINT('Ctrl Pts',(3.90000112250675,1.5728228815436,0.698773197673241));
#9970=CARTESIAN_POINT('Ctrl Pts',(3.90000049100668,1.56777898966077,0.699580906164169));
#9971=CARTESIAN_POINT('Ctrl Pts',(3.89999999374416,1.56266934880282,0.69999999924861));
#9972=CARTESIAN_POINT('Ctrl Pts',(3.89999999700315,1.55753217437,0.7));
#9973=CARTESIAN_POINT('Ctrl Pts',(3.9,1.68995649764597,0.));
#9974=CARTESIAN_POINT('Ctrl Pts',(3.9,1.68454744095908,0.101111134163871));
#9975=CARTESIAN_POINT('Ctrl Pts',(3.9,1.67913787721413,0.202223216861756));
#9976=CARTESIAN_POINT('Ctrl Pts',(3.9,1.66834172806373,0.404000675610066));
#9977=CARTESIAN_POINT('Ctrl Pts',(3.9,1.66295504272671,0.504667995047933));
#9978=CARTESIAN_POINT('Ctrl Pts',(3.9,1.657567947596,0.605334330700044));
#9979=CARTESIAN_POINT('Ctrl Pts',(3.90000000000029,-1.68995649764598,2.25514051876985E-17));
#9980=CARTESIAN_POINT('Ctrl Pts',(3.90375240214247,-1.67935614215062,0.202290156525516));
#9981=CARTESIAN_POINT('Ctrl Pts',(3.90750491350916,-1.66875579641967,0.404580311547879));
#9982=CARTESIAN_POINT('Ctrl Pts',(3.91125753584366,-1.65815546066147,0.606870465045848));
#9983=CARTESIAN_POINT('Ctrl Pts',(2.95719731373254,-1.63434162994996,-0.000186284957671625));
#9984=CARTESIAN_POINT('Ctrl Pts',(2.96263618266967,-1.62374249289717,0.202103577800055));
#9985=CARTESIAN_POINT('Ctrl Pts',(2.96807524459186,-1.6131433886527,0.404393433349269));
#9986=CARTESIAN_POINT('Ctrl Pts',(2.97351444051957,-1.60254429060724,0.606683290324339));
#9987=CARTESIAN_POINT('Ctrl Pts',(2.0151035222252,-1.5373601393942,-0.000515615972119944));
#9988=CARTESIAN_POINT('Ctrl Pts',(2.0222299762717,-1.52676329064944,0.20177372753372));
#9989=CARTESIAN_POINT('Ctrl Pts',(2.02935668076532,-1.51616649670304,0.404063061036967));
#9990=CARTESIAN_POINT('Ctrl Pts',(2.03648357820815,-1.50556972342972,0.606352393906678));
#9991=CARTESIAN_POINT('Ctrl Pts',(1.07355614839761,-1.3885225322474,-0.00102014041634142));
#9992=CARTESIAN_POINT('Ctrl Pts',(1.08237048982668,-1.37792954541675,0.201268457136957));
#9993=CARTESIAN_POINT('Ctrl Pts',(1.09118510562603,-1.36733662501784,0.403557046289628));
#9994=CARTESIAN_POINT('Ctrl Pts',(1.09999999998551,-1.35674377243019,0.605845626932519));
#9995=CARTESIAN_POINT('Ctrl Pts',(1.10000000359112,-1.35674374984279,0.605845627045242));
#9996=CARTESIAN_POINT('Ctrl Pts',(2.02777573897866,-1.50422778688462,0.60559460123127));
#9997=CARTESIAN_POINT('Ctrl Pts',(2.96295221054883,-1.60165319397541,0.605428415101273));
#9998=CARTESIAN_POINT('Ctrl Pts',(3.9,-1.657567947596,0.605334330700044));
#9999=CARTESIAN_POINT('Ctrl Pts',(3.90594750914669,-1.55788759822396,0.7));
#10000=CARTESIAN_POINT('Ctrl Pts',(2.96654482017732,-1.50183737247472,0.7));
#10001=CARTESIAN_POINT('Ctrl Pts',(2.02939151553635,-1.40396309164617,0.7));
#10002=CARTESIAN_POINT('Ctrl Pts',(1.1,-1.25565664448621,0.7));
#10003=CARTESIAN_POINT('Ctrl Pts',(3.90422602671531,-1.58673967158186,0.7));
#10004=CARTESIAN_POINT('Ctrl Pts',(2.9639697519154,-1.53062009474021,0.699999324449154));
#10005=CARTESIAN_POINT('Ctrl Pts',(2.02587169016863,-1.43262076012027,0.700001792708215));
#10006=CARTESIAN_POINT('Ctrl Pts',(1.09546090287069,-1.28410178925883,0.700000000000001));
#10007=CARTESIAN_POINT('Ctrl Pts',(3.90124198563808,-1.6367522482393,0.676652244116846));
#10008=CARTESIAN_POINT('Ctrl Pts',(2.95951584878018,-1.58051528054544,0.676683243227538));
#10009=CARTESIAN_POINT('Ctrl Pts',(2.01975879699698,-1.48229505764113,0.676737195552829));
#10010=CARTESIAN_POINT('Ctrl Pts',(1.08759175402576,-1.33341535796084,0.676819902351873));
#10011=CARTESIAN_POINT('Ctrl Pts',(3.90006887217438,-1.65641364884095,0.626981005337021));
#10012=CARTESIAN_POINT('Ctrl Pts',(2.95775794493813,-1.6001648299169,0.627061170854983));
#10013=CARTESIAN_POINT('Ctrl Pts',(2.01735267249256,-1.50192280897576,0.627202240820629));
#10014=CARTESIAN_POINT('Ctrl Pts',(1.08446813262788,-1.35299014570964,0.627416665943555));
#10015=CARTESIAN_POINT('Ctrl Pts',(3.9,-1.657567947596,0.605334330700044));
#10016=CARTESIAN_POINT('Ctrl Pts',(2.95765589353472,-1.60133715645388,0.605428946878649));
#10017=CARTESIAN_POINT('Ctrl Pts',(2.01720431860088,-1.50312513840151,0.605596482146283));
#10018=CARTESIAN_POINT('Ctrl Pts',(1.0842689834292,-1.35423815332579,0.605849891671036));
#10019=CARTESIAN_POINT('Ctrl Pts',(3.89999999700313,-1.55753217437,0.7));
#10020=CARTESIAN_POINT('Ctrl Pts',(2.96258932077475,-1.50142404037792,0.7));
#10021=CARTESIAN_POINT('Ctrl Pts',(2.02743012901897,-1.40365010593343,0.7));
#10022=CARTESIAN_POINT('Ctrl Pts',(1.1,-1.25565664448621,0.7));
#10023=CARTESIAN_POINT('Origin',(6.08012166120517,1.06778195214465E-16,
0.7));
#10024=CARTESIAN_POINT('Ctrl Pts',(1.1,1.25565664448621,0.7));
#10025=CARTESIAN_POINT('Ctrl Pts',(2.02743012901899,1.40365010593344,0.7));
#10026=CARTESIAN_POINT('Ctrl Pts',(2.96258932077472,1.50142404037792,0.7));
#10027=CARTESIAN_POINT('Ctrl Pts',(3.89999999700315,1.55753217437,0.7));
#10028=CARTESIAN_POINT('Ctrl Pts',(1.1,1.25565664448621,0.7));
#10029=CARTESIAN_POINT('Ctrl Pts',(2.02939151553637,1.40396309164617,0.7));
#10030=CARTESIAN_POINT('Ctrl Pts',(2.96654482017727,1.50183737247472,0.7));
#10031=CARTESIAN_POINT('Ctrl Pts',(3.90594750914669,1.55788759822396,0.7));
#10032=CARTESIAN_POINT('Ctrl Pts',(1.09546090287069,1.28410178925883,0.700000000000001));
#10033=CARTESIAN_POINT('Ctrl Pts',(2.02587169016866,1.43262076012027,0.700001792708215));
#10034=CARTESIAN_POINT('Ctrl Pts',(2.96396975191535,1.53062009474021,0.699999324449154));
#10035=CARTESIAN_POINT('Ctrl Pts',(3.90422602671531,1.58673967158186,0.7));
#10036=CARTESIAN_POINT('Ctrl Pts',(1.08759175402576,1.33341535796084,0.676819902351873));
#10037=CARTESIAN_POINT('Ctrl Pts',(2.019758796997,1.48229505764113,0.676737195552829));
#10038=CARTESIAN_POINT('Ctrl Pts',(2.95951584878014,1.58051528054544,0.676683243227538));
#10039=CARTESIAN_POINT('Ctrl Pts',(3.90124198563808,1.6367522482393,0.676652244116846));
#10040=CARTESIAN_POINT('Ctrl Pts',(1.08446813262788,1.35299014570964,0.627416665943555));
#10041=CARTESIAN_POINT('Ctrl Pts',(2.01735267249258,1.50192280897576,0.627202240820629));
#10042=CARTESIAN_POINT('Ctrl Pts',(2.95775794493809,1.6001648299169,0.627061170854983));
#10043=CARTESIAN_POINT('Ctrl Pts',(3.90006887217438,1.65641364884095,0.626981005337021));
#10044=CARTESIAN_POINT('Ctrl Pts',(1.0842689834292,1.35423815332579,0.605849891671036));
#10045=CARTESIAN_POINT('Ctrl Pts',(2.0172043186009,1.50312513840152,0.605596482146283));
#10046=CARTESIAN_POINT('Ctrl Pts',(2.95765589353468,1.60133715645387,0.605428946878649));
#10047=CARTESIAN_POINT('Ctrl Pts',(3.9,1.657567947596,0.605334330700044));
#10048=CARTESIAN_POINT('Ctrl Pts',(3.9,1.657567947596,0.605334330700044));
#10049=CARTESIAN_POINT('Ctrl Pts',(2.96295221054879,1.60165319397541,0.605428415101273));
#10050=CARTESIAN_POINT('Ctrl Pts',(2.02777573897867,1.50422778688462,0.60559460123127));
#10051=CARTESIAN_POINT('Ctrl Pts',(1.10000000359111,1.35674374984279,0.605845627045242));
#10052=CARTESIAN_POINT('Ctrl Pts',(1.07355614839761,1.3885225322474,-0.00102014041634139));
#10053=CARTESIAN_POINT('Ctrl Pts',(1.08237048982668,1.37792954541676,0.201268457136957));
#10054=CARTESIAN_POINT('Ctrl Pts',(1.09118510562602,1.36733662501784,0.403557046289628));
#10055=CARTESIAN_POINT('Ctrl Pts',(1.09999999998551,1.35674377243019,0.605845626932519));
#10056=CARTESIAN_POINT('Ctrl Pts',(2.0151035222252,1.5373601393942,-0.000515615972119942));
#10057=CARTESIAN_POINT('Ctrl Pts',(2.0222299762717,1.52676329064944,0.201773727533721));
#10058=CARTESIAN_POINT('Ctrl Pts',(2.02935668076532,1.51616649670304,0.404063061036968));
#10059=CARTESIAN_POINT('Ctrl Pts',(2.03648357820815,1.50556972342972,0.606352393906678));
#10060=CARTESIAN_POINT('Ctrl Pts',(2.95719731373254,1.63434162994996,-0.000186284957671606));
#10061=CARTESIAN_POINT('Ctrl Pts',(2.96263618266967,1.62374249289717,0.202103577800055));
#10062=CARTESIAN_POINT('Ctrl Pts',(2.96807524459186,1.6131433886527,0.404393433349269));
#10063=CARTESIAN_POINT('Ctrl Pts',(2.97351444051957,1.60254429060724,0.60668329032434));
#10064=CARTESIAN_POINT('Ctrl Pts',(3.90000000000029,1.68995649764598,4.33680868994202E-17));
#10065=CARTESIAN_POINT('Ctrl Pts',(3.90375240214247,1.67935614215062,0.202290156525516));
#10066=CARTESIAN_POINT('Ctrl Pts',(3.90750491350917,1.66875579641967,0.404580311547879));
#10067=CARTESIAN_POINT('Ctrl Pts',(3.91125753584366,1.65815546066147,0.606870465045848));
#10068=CARTESIAN_POINT('Origin',(0.9,1.44962962962963,0.));
#10069=CARTESIAN_POINT('',(0.900000000000025,-1.32415632515176,0.605901073595307));
#10070=CARTESIAN_POINT('Ctrl Pts',(0.900000000000025,-1.32415632515176,
0.605901073595307));
#10071=CARTESIAN_POINT('Ctrl Pts',(0.900000000000025,-1.33021622058432,
0.504787384877132));
#10072=CARTESIAN_POINT('Ctrl Pts',(0.900000000000001,-1.33627289299046,
0.403672458220672));
#10073=CARTESIAN_POINT('Ctrl Pts',(0.900000000000001,-1.3483639425303,0.201706128802639));
#10074=CARTESIAN_POINT('Ctrl Pts',(0.9,-1.3543984610184,0.100852646477479));
#10075=CARTESIAN_POINT('Ctrl Pts',(0.9,-1.3604297237941,0.));
#10076=CARTESIAN_POINT('',(0.9,-1.22294421121193,0.7));
#10077=CARTESIAN_POINT('Ctrl Pts',(0.899999998934589,-1.2229442093848,0.7));
#10078=CARTESIAN_POINT('Ctrl Pts',(0.89999998269596,-1.2309559991361,0.699999991698178));
#10079=CARTESIAN_POINT('Ctrl Pts',(0.900003161357076,-1.2389110096839,0.699008412490225));
#10080=CARTESIAN_POINT('Ctrl Pts',(0.900005837532895,-1.24666554379878,
0.697120920272419));
#10081=CARTESIAN_POINT('Ctrl Pts',(0.900007138246235,-1.25043451364619,
0.69620353424371));
#10082=CARTESIAN_POINT('Ctrl Pts',(0.900008321383585,-1.25415610217771,
0.695073675615989));
#10083=CARTESIAN_POINT('Ctrl Pts',(0.900009136546862,-1.25781268161099,
0.69373809091454));
#10084=CARTESIAN_POINT('Ctrl Pts',(0.90001081442992,-1.26533916477404,0.690989003700189));
#10085=CARTESIAN_POINT('Ctrl Pts',(0.900010659344479,-1.27251458345821,
0.687399440976464));
#10086=CARTESIAN_POINT('Ctrl Pts',(0.900008585023094,-1.27919110928202,
0.68304500924512));
#10087=CARTESIAN_POINT('Ctrl Pts',(0.900007251085311,-1.28348459539356,
0.680244796581297));
#10088=CARTESIAN_POINT('Ctrl Pts',(0.900005156998288,-1.28757155292352,
0.67712723751572));
#10089=CARTESIAN_POINT('Ctrl Pts',(0.900003422242992,-1.29140570811059,
0.673703384872626));
#10090=CARTESIAN_POINT('Ctrl Pts',(0.90000203719427,-1.29446694202502,0.670969741262059));
#10091=CARTESIAN_POINT('Ctrl Pts',(0.90000088611098,-1.29734878548314,0.668056850549005));
#10092=CARTESIAN_POINT('Ctrl Pts',(0.900000936626746,-1.30003070819003,
0.664973821719563));
#10093=CARTESIAN_POINT('Ctrl Pts',(0.90000103432908,-1.30521780373233,0.659010948495488));
#10094=CARTESIAN_POINT('Ctrl Pts',(0.900005119671874,-1.30966005175478,
0.652412896960716));
#10095=CARTESIAN_POINT('Ctrl Pts',(0.900006662646281,-1.31329014967729,
0.64534035177384));
#10096=CARTESIAN_POINT('Ctrl Pts',(0.900006837929091,-1.31370253096037,
0.644536906434065));
#10097=CARTESIAN_POINT('Ctrl Pts',(0.900006988901759,-1.3141043809937,0.64372731654354));
#10098=CARTESIAN_POINT('Ctrl Pts',(0.900007112770807,-1.31449556093743,
0.642911804846506));
#10099=CARTESIAN_POINT('Ctrl Pts',(0.900008198175579,-1.31792328224658,
0.635765868899185));
#10100=CARTESIAN_POINT('Ctrl Pts',(0.900006415208278,-1.32049402672979,
0.628253543462219));
#10101=CARTESIAN_POINT('Ctrl Pts',(0.900003664797616,-1.32215034643222,
0.620540220943237));
#10102=CARTESIAN_POINT('Ctrl Pts',(0.900001948338234,-1.32318401225236,
0.615726538031782));
#10103=CARTESIAN_POINT('Ctrl Pts',(0.900000000000001,-1.32386068836271,
0.610833984830158));
#10104=CARTESIAN_POINT('Ctrl Pts',(0.900000000000001,-1.32415632515176,
0.605901073595307));
#10105=CARTESIAN_POINT('',(0.9,1.22294421121193,0.7));
#10106=CARTESIAN_POINT('',(0.9,0.724814814814815,0.7));
#10107=CARTESIAN_POINT('',(0.900000000000027,1.32415632515176,0.605901073595307));
#10108=CARTESIAN_POINT('Ctrl Pts',(0.900000000000001,1.32415632515176,0.605901073595307));
#10109=CARTESIAN_POINT('Ctrl Pts',(0.900000000000001,1.32368299187747,0.613798977756921));
#10110=CARTESIAN_POINT('Ctrl Pts',(0.900004523569871,1.32223544152535,0.621596324701597));
#10111=CARTESIAN_POINT('Ctrl Pts',(0.900006356724635,1.31990036466821,0.629134362570908));
#10112=CARTESIAN_POINT('Ctrl Pts',(0.900007328861843,1.3186620540024,0.633131846706937));
#10113=CARTESIAN_POINT('Ctrl Pts',(0.900007702029268,1.31717322147439,0.637056437951431));
#10114=CARTESIAN_POINT('Ctrl Pts',(0.900007358328755,1.31544117393516,0.640882963165587));
#10115=CARTESIAN_POINT('Ctrl Pts',(0.900006707239278,1.31216006761937,0.648131745755711));
#10116=CARTESIAN_POINT('Ctrl Pts',(0.900003091243194,1.3080468004769,0.654946293188228));
#10117=CARTESIAN_POINT('Ctrl Pts',(0.900001489347898,1.30317324258861,0.661167512355852));
#10118=CARTESIAN_POINT('Ctrl Pts',(0.900001155878064,1.30215870403359,0.662462596327245));
#10119=CARTESIAN_POINT('Ctrl Pts',(0.90000093695446,1.30111105636563,0.663731893727214));
#10120=CARTESIAN_POINT('Ctrl Pts',(0.90000091848414,1.30003070515708,0.664973821721807));
#10121=CARTESIAN_POINT('Ctrl Pts',(0.90000089007412,1.29836896897911,0.666884086330845));
#10122=CARTESIAN_POINT('Ctrl Pts',(0.900001333486324,1.29662987445651,0.668729618924651));
#10123=CARTESIAN_POINT('Ctrl Pts',(0.900001997973453,1.2948182721625,0.670508241825176));
#10124=CARTESIAN_POINT('Ctrl Pts',(0.900004083621534,1.28913213515815,0.676090865298813));
#10125=CARTESIAN_POINT('Ctrl Pts',(0.900007925915178,1.28279871831387,0.680954424681199));
#10126=CARTESIAN_POINT('Ctrl Pts',(0.900009431597099,1.27598654051802,0.685053039288488));
#10127=CARTESIAN_POINT('Ctrl Pts',(0.900010426918848,1.2714833923965,0.687762403198649));
#10128=CARTESIAN_POINT('Ctrl Pts',(0.900010579450444,1.26676996242859,0.690136867340003));
#10129=CARTESIAN_POINT('Ctrl Pts',(0.900009885932263,1.26188774903006,0.692153145632694));
#10130=CARTESIAN_POINT('Ctrl Pts',(0.900008832351734,1.25447077696631,0.695216239878874));
#10131=CARTESIAN_POINT('Ctrl Pts',(0.900005746465811,1.24674633448708,0.697421320974322));
#10132=CARTESIAN_POINT('Ctrl Pts',(0.900003140090462,1.23886595492982,0.6987028844583));
#10133=CARTESIAN_POINT('Ctrl Pts',(0.900001403206082,1.23361448254879,0.699556916322089));
#10134=CARTESIAN_POINT('Ctrl Pts',(0.899999988093253,1.22829309040712,0.699999994457486));
#10135=CARTESIAN_POINT('Ctrl Pts',(0.899999998934588,1.2229442093848,0.7));
#10136=CARTESIAN_POINT('Ctrl Pts',(0.9,1.3604297237941,0.));
#10137=CARTESIAN_POINT('Ctrl Pts',(0.9,1.35439838926384,0.100853846331769));
#10138=CARTESIAN_POINT('Ctrl Pts',(0.9,1.34836379894337,0.201708528537181));
#10139=CARTESIAN_POINT('Ctrl Pts',(0.9,1.33627274925098,0.403674857922336));
#10140=CARTESIAN_POINT('Ctrl Pts',(0.900000000000027,1.33021614867672,0.504788584706939));
#10141=CARTESIAN_POINT('Ctrl Pts',(0.900000000000027,1.32415632515176,0.605901073595307));
#10142=CARTESIAN_POINT('Ctrl Pts',(0.900000000000001,-1.3604297237941,-1.73472347597681E-18));
#10143=CARTESIAN_POINT('Ctrl Pts',(0.909119345746934,-1.34984469470005,
0.202150401646216));
#10144=CARTESIAN_POINT('Ctrl Pts',(0.918238975454288,-1.33925973741039,
0.404300794324169));
#10145=CARTESIAN_POINT('Ctrl Pts',(0.92735889343571,-1.32867485341111,0.606451177918334));
#10146=CARTESIAN_POINT('Ctrl Pts',(0.693791632045388,-1.32642527651154,
-0.000115194085079675));
#10147=CARTESIAN_POINT('Ctrl Pts',(0.703280422539661,-1.31584113310577,
0.202035038813999));
#10148=CARTESIAN_POINT('Ctrl Pts',(0.712769508818954,-1.30525706820637,
0.404185262036053));
#10149=CARTESIAN_POINT('Ctrl Pts',(0.722258895242942,-1.29467308328318,
0.606335475483814));
#10150=CARTESIAN_POINT('Ctrl Pts',(0.487608314405001,-1.28990207050556,
-0.000238777108575344));
#10151=CARTESIAN_POINT('Ctrl Pts',(0.497466558273561,-1.27931888757273,
0.201911276725417));
#10152=CARTESIAN_POINT('Ctrl Pts',(0.507325109482935,-1.26873579028159,
0.404061320158324));
#10153=CARTESIAN_POINT('Ctrl Pts',(0.517183972542757,-1.25815278023897,
0.606211353085106));
#10154=CARTESIAN_POINT('Ctrl Pts',(0.281447431601629,-1.2507496025167,-0.000370926150909055));
#10155=CARTESIAN_POINT('Ctrl Pts',(0.291675125201343,-1.24016745708839,
0.201778938960696));
#10156=CARTESIAN_POINT('Ctrl Pts',(0.301903137322998,-1.2295854048496,0.403928792940867));
#10157=CARTESIAN_POINT('Ctrl Pts',(0.312131472716966,-1.21900344770756,
0.606078635650713));
#10158=CARTESIAN_POINT('',(0.313137632044026,-1.21919552599285,0.606079286803921));
#10159=CARTESIAN_POINT('Ctrl Pts',(0.28146619846596,-1.25073018526678,-6.36968776335234E-17));
#10160=CARTESIAN_POINT('Ctrl Pts',(0.292023490345879,-1.2402182973453,0.20202640462578));
#10161=CARTESIAN_POINT('Ctrl Pts',(0.302580635585432,-1.22970674279184,
0.404052833452346));
#10162=CARTESIAN_POINT('Ctrl Pts',(0.313137632044028,-1.21919552599286,
0.606079286803922));
#10163=CARTESIAN_POINT('Ctrl Pts',(0.313137632044026,-1.21919552599285,
0.606079286803921));
#10164=CARTESIAN_POINT('Ctrl Pts',(0.508347756773358,-1.25646926692181,
0.606016122348466));
#10165=CARTESIAN_POINT('Ctrl Pts',(0.703992099548353,-1.29143758865737,
0.605956720831638));
#10166=CARTESIAN_POINT('Ctrl Pts',(0.900000000000031,-1.32415632515176,
0.605901073595307));
#10167=CARTESIAN_POINT('Ctrl Pts',(0.916434425702686,-1.22569269236154,
0.7));
#10168=CARTESIAN_POINT('Ctrl Pts',(0.72117838049967,-1.193102781986,0.7));
#10169=CARTESIAN_POINT('Ctrl Pts',(0.526295996270969,-1.15827411715321,
0.7));
#10170=CARTESIAN_POINT('Ctrl Pts',(0.3318563713692,-1.12115139781564,0.7));
#10171=CARTESIAN_POINT('Ctrl Pts',(0.911693828447622,-1.25409504944868,
0.700000000000001));
#10172=CARTESIAN_POINT('Ctrl Pts',(0.716221724293519,-1.22145811194286,
0.699999606692487));
#10173=CARTESIAN_POINT('Ctrl Pts',(0.52112301919326,-1.18657973614434,0.700000445015345));
#10174=CARTESIAN_POINT('Ctrl Pts',(0.32646265058614,-1.14940237362229,0.699999999999999));
#10175=CARTESIAN_POINT('Ctrl Pts',(0.903473253113197,-1.30334701150065,
0.676847307332805));
#10176=CARTESIAN_POINT('Ctrl Pts',(0.707628846166824,-1.27063023858114,
0.676865462359186));
#10177=CARTESIAN_POINT('Ctrl Pts',(0.512149925983835,-1.23566412474798,
0.676884474751893));
#10178=CARTESIAN_POINT('Ctrl Pts',(0.317109102097966,-1.19839394783867,
0.676905055067496));
#10179=CARTESIAN_POINT('Ctrl Pts',(0.900209809599689,-1.32289929215588,
0.627459885485154));
#10180=CARTESIAN_POINT('Ctrl Pts',(0.704212910592823,-1.29017057588713,
0.627506965865002));
#10181=CARTESIAN_POINT('Ctrl Pts',(0.50858160780484,-1.25519230329596,0.627556915196293));
#10182=CARTESIAN_POINT('Ctrl Pts',(0.31338355686088,-1.21790743260971,0.627610331402299));
#10183=CARTESIAN_POINT('Ctrl Pts',(0.900000000000031,-1.32415632515176,
0.605901073595307));
#10184=CARTESIAN_POINT('Ctrl Pts',(0.703992099548353,-1.29143758865737,
0.605956720831638));
#10185=CARTESIAN_POINT('Ctrl Pts',(0.508347756773358,-1.25646926692181,
0.606016122348466));
#10186=CARTESIAN_POINT('Ctrl Pts',(0.313137632044026,-1.21919552599285,
0.606079286803921));
#10187=CARTESIAN_POINT('',(0.3318563713692,-1.12115139781563,0.7));
#10188=CARTESIAN_POINT('Origin',(0.331856371369202,-1.12115139781563,0.6));
#10189=CARTESIAN_POINT('Ctrl Pts',(0.899999998934586,-1.2229442093848,0.7));
#10190=CARTESIAN_POINT('Ctrl Pts',(0.71024282334811,-1.19114655107378,0.7));
#10191=CARTESIAN_POINT('Ctrl Pts',(0.520840466228891,-1.15723253876768,
0.7));
#10192=CARTESIAN_POINT('Ctrl Pts',(0.3318563713692,-1.12115139781564,0.7));
#10193=CARTESIAN_POINT('Origin',(6.08012166120517,1.06778195214465E-16,
0.7));
#10194=CARTESIAN_POINT('',(0.331856371369203,1.12115139781563,0.7));
#10195=CARTESIAN_POINT('',(0.3318563713692,-0.7,0.7));
#10196=CARTESIAN_POINT('Ctrl Pts',(0.331856371369202,1.12115139781564,0.7));
#10197=CARTESIAN_POINT('Ctrl Pts',(0.520840466228894,1.15723253876768,0.7));
#10198=CARTESIAN_POINT('Ctrl Pts',(0.710242823348114,1.19114655107378,0.7));
#10199=CARTESIAN_POINT('Ctrl Pts',(0.899999998934589,1.2229442093848,0.7));
#10200=CARTESIAN_POINT('Ctrl Pts',(0.281447431601628,1.2507496025167,-0.000370926150909064));
#10201=CARTESIAN_POINT('Ctrl Pts',(0.291675125201342,1.24016745708839,0.201778938960695));
#10202=CARTESIAN_POINT('Ctrl Pts',(0.301903137322998,1.2295854048496,0.403928792940867));
#10203=CARTESIAN_POINT('Ctrl Pts',(0.312131472716965,1.21900344770756,0.606078635650713));
#10204=CARTESIAN_POINT('Ctrl Pts',(0.487608314405001,1.28990207050556,-0.000238777108575355));
#10205=CARTESIAN_POINT('Ctrl Pts',(0.497466558273561,1.27931888757273,0.201911276725417));
#10206=CARTESIAN_POINT('Ctrl Pts',(0.507325109482935,1.26873579028159,0.404061320158324));
#10207=CARTESIAN_POINT('Ctrl Pts',(0.517183972542757,1.25815278023897,0.606211353085106));
#10208=CARTESIAN_POINT('Ctrl Pts',(0.693791632045388,1.32642527651154,-0.000115194085079627));
#10209=CARTESIAN_POINT('Ctrl Pts',(0.703280422539661,1.31584113310577,0.202035038813999));
#10210=CARTESIAN_POINT('Ctrl Pts',(0.712769508818955,1.30525706820637,0.404185262036054));
#10211=CARTESIAN_POINT('Ctrl Pts',(0.722258895242942,1.29467308328318,0.606335475483814));
#10212=CARTESIAN_POINT('Ctrl Pts',(0.900000000000002,1.3604297237941,4.33680868994202E-17));
#10213=CARTESIAN_POINT('Ctrl Pts',(0.909119345746935,1.34984469470005,0.202150401646216));
#10214=CARTESIAN_POINT('Ctrl Pts',(0.918238975454289,1.33925973741039,0.40430079432417));
#10215=CARTESIAN_POINT('Ctrl Pts',(0.927358893435711,1.32867485341111,0.606451177918334));
#10216=CARTESIAN_POINT('',(0.313137632044028,1.21919552599286,0.606079286803921));
#10217=CARTESIAN_POINT('Ctrl Pts',(0.900000000000026,1.32415632515176,0.605901073595307));
#10218=CARTESIAN_POINT('Ctrl Pts',(0.703992099548352,1.29143758865737,0.605956720831638));
#10219=CARTESIAN_POINT('Ctrl Pts',(0.508347756773358,1.25646926692181,0.606016122348466));
#10220=CARTESIAN_POINT('Ctrl Pts',(0.313137632044028,1.21919552599286,0.606079286803921));
#10221=CARTESIAN_POINT('Ctrl Pts',(0.313137632044028,1.21919552599286,0.606079286803922));
#10222=CARTESIAN_POINT('Ctrl Pts',(0.302580635585432,1.22970674279184,0.404052833452346));
#10223=CARTESIAN_POINT('Ctrl Pts',(0.29202349034588,1.2402182973453,0.20202640462578));
#10224=CARTESIAN_POINT('Ctrl Pts',(0.28146619846596,1.25073018526678,-6.5594231435373E-18));
#10225=CARTESIAN_POINT('Ctrl Pts',(0.331856371369202,1.12115139781564,0.7));
#10226=CARTESIAN_POINT('Ctrl Pts',(0.526295996270969,1.15827411715321,0.7));
#10227=CARTESIAN_POINT('Ctrl Pts',(0.72117838049967,1.193102781986,0.7));
#10228=CARTESIAN_POINT('Ctrl Pts',(0.916434425702682,1.22569269236154,0.7));
#10229=CARTESIAN_POINT('Ctrl Pts',(0.326462650586141,1.14940237362229,0.699999999999999));
#10230=CARTESIAN_POINT('Ctrl Pts',(0.52112301919326,1.18657973614434,0.700000445015345));
#10231=CARTESIAN_POINT('Ctrl Pts',(0.716221724293519,1.22145811194286,0.699999606692487));
#10232=CARTESIAN_POINT('Ctrl Pts',(0.911693828447618,1.25409504944868,0.700000000000001));
#10233=CARTESIAN_POINT('Ctrl Pts',(0.317109102097967,1.19839394783867,0.676905055067496));
#10234=CARTESIAN_POINT('Ctrl Pts',(0.512149925983836,1.23566412474798,0.676884474751893));
#10235=CARTESIAN_POINT('Ctrl Pts',(0.707628846166824,1.27063023858114,0.676865462359185));
#10236=CARTESIAN_POINT('Ctrl Pts',(0.903473253113193,1.30334701150065,0.676847307332805));
#10237=CARTESIAN_POINT('Ctrl Pts',(0.313383556860882,1.21790743260971,0.627610331402299));
#10238=CARTESIAN_POINT('Ctrl Pts',(0.508581607804839,1.25519230329596,0.627556915196293));
#10239=CARTESIAN_POINT('Ctrl Pts',(0.704212910592822,1.29017057588713,0.627506965865002));
#10240=CARTESIAN_POINT('Ctrl Pts',(0.900209809599685,1.32289929215587,0.627459885485154));
#10241=CARTESIAN_POINT('Ctrl Pts',(0.313137632044028,1.21919552599286,0.606079286803921));
#10242=CARTESIAN_POINT('Ctrl Pts',(0.508347756773358,1.25646926692181,0.606016122348466));
#10243=CARTESIAN_POINT('Ctrl Pts',(0.703992099548352,1.29143758865737,0.605956720831638));
#10244=CARTESIAN_POINT('Ctrl Pts',(0.900000000000026,1.32415632515176,0.605901073595307));
#10245=CARTESIAN_POINT('Origin',(0.3318563713692,1.12115139781563,0.6));
#10246=CARTESIAN_POINT('Origin',(0.3318563713692,1.12115139781563,0.6));
#10247=CARTESIAN_POINT('Origin',(0.3318563713692,1.12115139781563,0.6));
#10248=CARTESIAN_POINT('Origin',(0.331856371369201,1.12115139781563,0.6));
#10249=CARTESIAN_POINT('Origin',(11.6681436286308,1.2964346619681,0.6));
#10250=CARTESIAN_POINT('Origin',(11.6681436286308,1.2964346619681,0.6));
#10251=CARTESIAN_POINT('',(11.7680065821063,1.2964346619681,0.605233595624295));
#10252=CARTESIAN_POINT('Origin',(11.6681436286308,1.2964346619681,0.6));
#10253=CARTESIAN_POINT('Origin',(11.6681436286308,1.2964346619681,0.6));
#10254=CARTESIAN_POINT('Origin',(0.3318563713692,-1.12115139781563,0.6));
#10255=CARTESIAN_POINT('Origin',(0.3318563713692,-1.12115139781563,0.6));
#10256=CARTESIAN_POINT('Origin',(0.3318563713692,-1.12115139781563,0.6));
#10257=CARTESIAN_POINT('Origin',(0.3318563713692,-0.7,0.6));
#10258=CARTESIAN_POINT('Ctrl Pts',(0.281398851089427,-1.25079724300364,
-0.00128877254616805));
#10259=CARTESIAN_POINT('Ctrl Pts',(0.291978592719145,-1.24026300108396,
0.201167222825305));
#10260=CARTESIAN_POINT('Ctrl Pts',(0.302558187088771,-1.2297290939422,0.403623242499903));
#10261=CARTESIAN_POINT('Ctrl Pts',(0.313137632044028,-1.21919552599286,
0.606079286803922));
#10262=CARTESIAN_POINT('Ctrl Pts',(0.258825925396095,-1.24645021448495,
-0.000331836826913007));
#10263=CARTESIAN_POINT('Ctrl Pts',(0.269412087408768,-1.23590982471973,
0.202123507634926));
#10264=CARTESIAN_POINT('Ctrl Pts',(0.279998097240749,-1.22537010804418,
0.404578894752494));
#10265=CARTESIAN_POINT('Ctrl Pts',(0.290584031570127,-1.21483034200885,
0.60703428203898));
#10266=CARTESIAN_POINT('Ctrl Pts',(0.216858515231733,-1.22156435206688,
0.000573427186746937));
#10267=CARTESIAN_POINT('Ctrl Pts',(0.22746089442761,-1.21102065820065,0.20302778119957));
#10268=CARTESIAN_POINT('Ctrl Pts',(0.238063405890532,-1.20047706879609,
0.405482132943502));
#10269=CARTESIAN_POINT('Ctrl Pts',(0.248665715176951,-1.18993398276804,
0.607936521147589));
#10270=CARTESIAN_POINT('Ctrl Pts',(0.20022524016831,-1.1757120364715,-0.000939345874739115));
#10271=CARTESIAN_POINT('Ctrl Pts',(0.210835545796271,-1.16517845930889,
0.201515175954065));
#10272=CARTESIAN_POINT('Ctrl Pts',(0.221445511453644,-1.15464532122135,
0.403969738345816));
#10273=CARTESIAN_POINT('Ctrl Pts',(0.232055819885544,-1.1441124535127,0.606424296559432));
#10274=CARTESIAN_POINT('Ctrl Pts',(0.200162791320387,-1.15273540576203,
-0.00213094087794781));
#10275=CARTESIAN_POINT('Ctrl Pts',(0.210772999146098,-1.14220702337553,
0.200323884929633));
#10276=CARTESIAN_POINT('Ctrl Pts',(0.221383207999129,-1.13167901896849,
0.402778730339676));
#10277=CARTESIAN_POINT('Ctrl Pts',(0.231993417893744,-1.12115139781563,
0.605233595624295));
#10278=CARTESIAN_POINT('Origin',(11.6681436286308,-1.2964346619681,0.6));
#10279=CARTESIAN_POINT('',(11.7680065821063,-1.2964346619681,0.605233595624295));
#10280=CARTESIAN_POINT('Origin',(11.6681436286308,-1.2964346619681,0.6));
#10281=CARTESIAN_POINT('Origin',(11.6681436286308,-1.2964346619681,0.6));
#10282=CARTESIAN_POINT('Origin',(11.6681436286308,0.8,0.6));
#10283=CARTESIAN_POINT('',(11.7680065821063,0.8,0.605233595624295));
#10284=CARTESIAN_POINT('Ctrl Pts',(11.7998406965532,-1.32812796269332,-0.00219749346969486));
#10285=CARTESIAN_POINT('Ctrl Pts',(11.7892293257052,-1.31756329650235,0.200279524124498));
#10286=CARTESIAN_POINT('Ctrl Pts',(11.778617954226,-1.30699886176745,0.402756553762325));
#10287=CARTESIAN_POINT('Ctrl Pts',(11.7680065821063,-1.2964346619681,0.605233595624295));
#10288=CARTESIAN_POINT('Ctrl Pts',(11.7997644051931,-1.35610429277321,-0.000741767599518841));
#10289=CARTESIAN_POINT('Ctrl Pts',(11.7891529352516,-1.34553639595159,0.201735054786578));
#10290=CARTESIAN_POINT('Ctrl Pts',(11.7785417923834,-1.33496887357233,0.404211913913734));
#10291=CARTESIAN_POINT('Ctrl Pts',(11.7679303202531,-1.32440140973518,0.606688758469115));
#10292=CARTESIAN_POINT('Ctrl Pts',(11.777798894316,-1.40464673224301,0.000639873095493681));
#10293=CARTESIAN_POINT('Ctrl Pts',(11.7671928076068,-1.39407357725403,0.203116666245104));
#10294=CARTESIAN_POINT('Ctrl Pts',(11.7565866683578,-1.38350056680667,0.405593463707878));
#10295=CARTESIAN_POINT('Ctrl Pts',(11.7459806329718,-1.37292778989405,0.608070278434593));
#10296=CARTESIAN_POINT('Ctrl Pts',(11.7305637688674,-1.42539741767755,-0.000752904078362463));
#10297=CARTESIAN_POINT('Ctrl Pts',(11.7199663219939,-1.4148278080644,0.201724510929383));
#10298=CARTESIAN_POINT('Ctrl Pts',(11.7093688723049,-1.40425849106451,0.404201940657439));
#10299=CARTESIAN_POINT('Ctrl Pts',(11.6987715660822,-1.39368929079062,0.606679383299034));
#10300=CARTESIAN_POINT('Ctrl Pts',(11.7096810564041,-1.4274931182575,-0.0017379730583696));
#10301=CARTESIAN_POINT('Ctrl Pts',(11.6990862989954,-1.41692678914967,0.200739752511227));
#10302=CARTESIAN_POINT('Ctrl Pts',(11.6884916259906,-1.40636067879325,0.403217493356832));
#10303=CARTESIAN_POINT('Ctrl Pts',(11.6778970386953,-1.39579479040469,0.605695249702977));
#10304=CARTESIAN_POINT('Ctrl Pts',(11.7997255308004,-1.32801330383774,1.58293517182884E-17));
#10305=CARTESIAN_POINT('Ctrl Pts',(11.7891525485321,-1.31748685893698,0.201744519857947));
#10306=CARTESIAN_POINT('Ctrl Pts',(11.7785795656372,-1.30696064383315,0.403489051673192));
#10307=CARTESIAN_POINT('Ctrl Pts',(11.7680065821063,-1.2964346619681,0.605233595624295));
#10308=CARTESIAN_POINT('Ctrl Pts',(11.7096782931395,1.42749036240749,-0.00168516396645821));
#10309=CARTESIAN_POINT('Ctrl Pts',(11.6990844568337,1.41692495195436,0.200774958575157));
#10310=CARTESIAN_POINT('Ctrl Pts',(11.6884907049172,1.40635976021489,0.403235096390144));
#10311=CARTESIAN_POINT('Ctrl Pts',(11.6778970386953,1.39579479040469,0.605695249702978));
#10312=CARTESIAN_POINT('Ctrl Pts',(11.7375219088137,1.42469609383707,-0.000371738767665111));
#10313=CARTESIAN_POINT('Ctrl Pts',(11.7269244310859,1.41412622652679,0.202087962343291));
#10314=CARTESIAN_POINT('Ctrl Pts',(11.7163270893473,1.40355692684423,0.404547700208143));
#10315=CARTESIAN_POINT('Ctrl Pts',(11.7057297418778,1.39298745758592,0.607007427831054));
#10316=CARTESIAN_POINT('Ctrl Pts',(11.7837126264455,1.39812338730171,0.000662527065309348));
#10317=CARTESIAN_POINT('Ctrl Pts',(11.7731059659782,1.38755170250994,0.203121672627585));
#10318=CARTESIAN_POINT('Ctrl Pts',(11.762499302106,1.37698011891703,0.405580822779681));
#10319=CARTESIAN_POINT('Ctrl Pts',(11.7518926781287,1.36640881816393,0.608039989525598));
#10320=CARTESIAN_POINT('Ctrl Pts',(11.7997807104374,1.34910745421534,-0.00105289019631603));
#10321=CARTESIAN_POINT('Ctrl Pts',(11.7891702365097,1.33854134055748,0.201406383632416));
#10322=CARTESIAN_POINT('Ctrl Pts',(11.7785598611315,1.32797539467558,0.403865671186622));
#10323=CARTESIAN_POINT('Ctrl Pts',(11.7679493857164,1.31740972279341,0.60632496775791));
#10324=CARTESIAN_POINT('Ctrl Pts',(11.7998379289556,1.32812520727701,-0.00214468456243374));
#10325=CARTESIAN_POINT('Ctrl Pts',(11.78922748064,1.31756145959839,0.200314730064766));
#10326=CARTESIAN_POINT('Ctrl Pts',(11.7786170316934,1.30699794333589,0.402774156733522));
#10327=CARTESIAN_POINT('Ctrl Pts',(11.7680065821063,1.2964346619681,0.605233595624295));
#10328=CARTESIAN_POINT('Ctrl Pts',(11.7680065821063,1.2964346619681,0.605233595624295));
#10329=CARTESIAN_POINT('Ctrl Pts',(11.7785795656372,1.30696064383315,0.403489051673192));
#10330=CARTESIAN_POINT('Ctrl Pts',(11.7891525485321,1.31748685893698,0.201744519857946));
#10331=CARTESIAN_POINT('Ctrl Pts',(11.7997255308004,1.32801330383774,3.10081821330854E-17));
#10332=CARTESIAN_POINT('Ctrl Pts',(11.3905090053564,1.32332268868375,0.7));
#10333=CARTESIAN_POINT('Ctrl Pts',(11.4830653488871,1.31448403714216,0.7));
#10334=CARTESIAN_POINT('Ctrl Pts',(11.5756099286391,1.3055179747114,0.7));
#10335=CARTESIAN_POINT('Ctrl Pts',(11.6681436286308,1.2964346619681,0.7));
#10336=CARTESIAN_POINT('Ctrl Pts',(11.3932507170007,1.35203326785047,0.7));
#10337=CARTESIAN_POINT('Ctrl Pts',(11.4858332859074,1.34318985044544,0.699999917777441));
#10338=CARTESIAN_POINT('Ctrl Pts',(11.5784027531871,1.33421922733773,0.700000082825348));
#10339=CARTESIAN_POINT('Ctrl Pts',(11.6709605510772,1.32513126902304,0.7));
#10340=CARTESIAN_POINT('Ctrl Pts',(11.3980029235658,1.40179729139028,0.67675176769038));
#10341=CARTESIAN_POINT('Ctrl Pts',(11.4906306781252,1.39294591144353,0.676755553516685));
#10342=CARTESIAN_POINT('Ctrl Pts',(11.583243842395,1.38396722707511,0.676759299309383));
#10343=CARTESIAN_POINT('Ctrl Pts',(11.6758431636759,1.37487151491717,0.676763114282959));
#10344=CARTESIAN_POINT('Ctrl Pts',(11.3998836071583,1.4214913811319,0.627256563056779));
#10345=CARTESIAN_POINT('Ctrl Pts',(11.4925297866457,1.41264104586547,0.627266369072496));
#10346=CARTESIAN_POINT('Ctrl Pts',(11.5851604051362,1.40366358810601,0.627276165220861));
#10347=CARTESIAN_POINT('Ctrl Pts',(11.6777767156198,1.39456903283364,0.627286048421068));
#10348=CARTESIAN_POINT('Ctrl Pts',(11.4,1.4227102204299,0.605660349289938));
#10349=CARTESIAN_POINT('Ctrl Pts',(11.4926474653491,1.41386220753305,0.605671932550561));
#10350=CARTESIAN_POINT('Ctrl Pts',(11.585279512325,1.40488700096013,0.605683574233495));
#10351=CARTESIAN_POINT('Ctrl Pts',(11.6778970386953,1.39579479040469,0.605695249702977));
#10352=CARTESIAN_POINT('Ctrl Pts',(0.200160078391861,1.15273809776858,-0.00218270663797729));
#10353=CARTESIAN_POINT('Ctrl Pts',(0.210771190526905,1.14220881798213,0.200289374419605));
#10354=CARTESIAN_POINT('Ctrl Pts',(0.221382303689445,1.13167991623912,0.402761475082968));
#10355=CARTESIAN_POINT('Ctrl Pts',(0.231993417893744,1.12115139781563,0.605233595624295));
#10356=CARTESIAN_POINT('Ctrl Pts',(0.200222527243758,1.17571472979894,-0.000991111558954063));
#10357=CARTESIAN_POINT('Ctrl Pts',(0.210833737189325,1.165180254798,0.201480665494204));
#10358=CARTESIAN_POINT('Ctrl Pts',(0.22144460713556,1.15464621893915,0.403952483115279));
#10359=CARTESIAN_POINT('Ctrl Pts',(0.232055819885544,1.1441124535127,0.606424296559433));
#10360=CARTESIAN_POINT('Ctrl Pts',(0.216855804290742,1.22156704800519,0.000521661548984882));
#10361=CARTESIAN_POINT('Ctrl Pts',(0.22745908713481,1.21102245544698,0.202993270772045));
#10362=CARTESIAN_POINT('Ctrl Pts',(0.238062502254218,1.2004779673848,0.405464877727456));
#10363=CARTESIAN_POINT('Ctrl Pts',(0.248665715176951,1.18993398276804,0.607936521147589));
#10364=CARTESIAN_POINT('Ctrl Pts',(0.258823218619159,1.24645290953083,-0.000383602721372307));
#10365=CARTESIAN_POINT('Ctrl Pts',(0.269410282911183,1.23591162135389,0.202088997034388));
#10366=CARTESIAN_POINT('Ctrl Pts',(0.279997195000074,1.22537100634993,0.404561639451295));
#10367=CARTESIAN_POINT('Ctrl Pts',(0.290584031570127,1.21483034200885,0.60703428203898));
#10368=CARTESIAN_POINT('Ctrl Pts',(0.281396145950812,1.25079993650842,-0.00134053860524368));
#10369=CARTESIAN_POINT('Ctrl Pts',(0.291976789318506,1.24026479669674,0.201132712115111));
#10370=CARTESIAN_POINT('Ctrl Pts',(0.302557285401186,1.22972999171968,0.403605987142707));
#10371=CARTESIAN_POINT('Ctrl Pts',(0.313137632044028,1.21919552599286,0.606079286803922));
#10372=CARTESIAN_POINT('Origin',(11.8002740930491,1.6,-0.0104671912485888));
#10373=CARTESIAN_POINT('Origin',(0.3318563713692,1.12115139781563,0.6));
#10374=CARTESIAN_POINT('',(0.331856371369203,1.12115139781563,0.9));
#10375=CARTESIAN_POINT('',(0.0322675109428288,1.12115139781563,0.615700786872883));
#10376=CARTESIAN_POINT('Origin',(0.3318563713692,1.12115139781563,0.6));
#10377=CARTESIAN_POINT('',(0.275700153393682,1.4152837823473,0.618237860411764));
#10378=CARTESIAN_POINT('Origin',(0.3318563713692,1.12115139781563,0.6));
#10379=CARTESIAN_POINT('Origin',(0.331856371369201,1.12115139781563,0.600000000000001));
#10380=CARTESIAN_POINT('Origin',(11.6681436286308,1.2964346619681,0.6));
#10381=CARTESIAN_POINT('',(11.6681436286308,1.2964346619681,0.9));
#10382=CARTESIAN_POINT('',(11.6974038588243,1.59451504727786,0.617085749108931));
#10383=CARTESIAN_POINT('Origin',(11.6681436286308,1.2964346619681,0.6));
#10384=CARTESIAN_POINT('',(11.9677324890572,1.2964346619681,0.615700786872884));
#10385=CARTESIAN_POINT('Origin',(11.6681436286308,1.2964346619681,0.6));
#10386=CARTESIAN_POINT('Origin',(11.6681436286308,1.2964346619681,0.6));
#10387=CARTESIAN_POINT('Origin',(0.3318563713692,-1.12115139781563,0.6));
#10388=CARTESIAN_POINT('',(0.3318563713692,-1.12115139781563,0.9));
#10389=CARTESIAN_POINT('',(0.27570015339368,-1.4152837823473,0.618237860411764));
#10390=CARTESIAN_POINT('Origin',(0.331856371369206,-1.12115139781563,0.6));
#10391=CARTESIAN_POINT('',(0.0322675109428289,-1.12115139781563,0.615700786872884));
#10392=CARTESIAN_POINT('Origin',(0.3318563713692,-1.12115139781563,0.6));
#10393=CARTESIAN_POINT('Origin',(0.331856371369201,-1.12115139781563,0.6));
#10394=CARTESIAN_POINT('Origin',(0.3318563713692,-0.7,0.6));
#10395=CARTESIAN_POINT('',(0.0322675109428288,-0.7,0.615700786872883));
#10396=CARTESIAN_POINT('',(0.3318563713692,-0.7,0.9));
#10397=CARTESIAN_POINT('Ctrl Pts',(0.243379792658812,-1.44768816351885,
-0.00386660544379547));
#10398=CARTESIAN_POINT('Ctrl Pts',(0.254153714020244,-1.43688644166428,
0.203501514337738));
#10399=CARTESIAN_POINT('Ctrl Pts',(0.264927169923045,-1.42608498030896,
0.410869669467268));
#10400=CARTESIAN_POINT('Ctrl Pts',(0.275700153393682,-1.4152837823473,0.618237860411764));
#10401=CARTESIAN_POINT('Ctrl Pts',(0.165985306518657,-1.43278556900406,
-0.000585522405354874));
#10402=CARTESIAN_POINT('Ctrl Pts',(0.176781886982148,-1.42196211044871,
0.206780297826791));
#10403=CARTESIAN_POINT('Ctrl Pts',(0.187577631459021,-1.41114055376332,
0.414146260476818));
#10404=CARTESIAN_POINT('Ctrl Pts',(0.198373523197449,-1.40031743725927,
0.621512129789107));
#10405=CARTESIAN_POINT('Ctrl Pts',(0.0420337764471552,-1.35067831466576,
0.00164062070145552));
#10406=CARTESIAN_POINT('Ctrl Pts',(0.0528811856485653,-1.33984924001505,
0.209003590924217));
#10407=CARTESIAN_POINT('Ctrl Pts',(0.0637288270387668,-1.3290196870647,
0.416366521726085));
#10408=CARTESIAN_POINT('Ctrl Pts',(0.0745760486629849,-1.31819094697801,
0.623729515932473));
#10409=CARTESIAN_POINT('Ctrl Pts',(-0.000174449685670057,-1.21258510413485,
-0.00332869829739982));
#10410=CARTESIAN_POINT('Ctrl Pts',(0.0106931634330696,-1.20178787588112,
0.204035045544629));
#10411=CARTESIAN_POINT('Ctrl Pts',(0.0215603573327632,-1.19099068058357,
0.411398812224037));
#10412=CARTESIAN_POINT('Ctrl Pts',(0.0324279732074593,-1.18019411246525,
0.618762589277523));
#10413=CARTESIAN_POINT('Ctrl Pts',(-0.000335035344191381,-1.15350137313465,
-0.00639285519773308));
#10414=CARTESIAN_POINT('Ctrl Pts',(0.0105324790023165,-1.1427176497384,
0.200971671503832));
#10415=CARTESIAN_POINT('Ctrl Pts',(0.0213999944262164,-1.13193432274319,
0.408336218763261));
#10416=CARTESIAN_POINT('Ctrl Pts',(0.0322675109428286,-1.12115139781563,
0.615700786872884));
#10417=CARTESIAN_POINT('Ctrl Pts',(0.243580684154575,-1.44748675362873,
-2.16840434497101E-17));
#10418=CARTESIAN_POINT('Ctrl Pts',(0.254287635915809,-1.43675217163244,
0.206079251738322));
#10419=CARTESIAN_POINT('Ctrl Pts',(0.264994127943615,-1.42601784692504,
0.412158538389471));
#10420=CARTESIAN_POINT('Ctrl Pts',(0.275700153393682,-1.4152837823473,0.618237860411764));
#10421=CARTESIAN_POINT('Ctrl Pts',(0.0322675109428286,-1.12115139781563,
0.615700786872884));
#10422=CARTESIAN_POINT('Ctrl Pts',(0.0215116728964671,-1.13182351356624,
0.410467170919192));
#10423=CARTESIAN_POINT('Ctrl Pts',(0.0107558359204751,-1.14249602316337,
0.205233575389367));
#10424=CARTESIAN_POINT('Ctrl Pts',(-1.41190227911925E-16,-1.15316892111333,
8.06646416329215E-17));
#10425=CARTESIAN_POINT('Origin',(11.6681436286308,-1.2964346619681,0.6));
#10426=CARTESIAN_POINT('',(11.9677324890572,-1.2964346619681,0.615700786872884));
#10427=CARTESIAN_POINT('',(11.6974038588243,-1.59451504727786,0.617085749108931));
#10428=CARTESIAN_POINT('Origin',(11.6681436286308,-1.2964346619681,0.600000000000001));
#10429=CARTESIAN_POINT('',(11.6681436286308,-1.2964346619681,0.9));
#10430=CARTESIAN_POINT('Origin',(11.6681436286308,-1.2964346619681,0.6));
#10431=CARTESIAN_POINT('Origin',(11.6681436286308,-1.2964346619681,0.6));
#10432=CARTESIAN_POINT('Origin',(11.6681436286308,0.8,0.6));
#10433=CARTESIAN_POINT('',(11.9677324890572,0.8,0.615700786872884));
#10434=CARTESIAN_POINT('',(11.6681436286308,0.8,0.9));
#10435=CARTESIAN_POINT('Ctrl Pts',(11.6681436286308,-1.2964346619681,0.9));
#10436=CARTESIAN_POINT('Ctrl Pts',(10.0505146497799,-1.45522470190849,0.9));
#10437=CARTESIAN_POINT('Ctrl Pts',(7.34698379851713,-1.66064017564263,0.9));
#10438=CARTESIAN_POINT('Ctrl Pts',(3.5507249968367,-1.5921338472202,0.9));
#10439=CARTESIAN_POINT('Ctrl Pts',(1.39628032950236,-1.32437289587156,0.9));
#10440=CARTESIAN_POINT('Ctrl Pts',(0.331856371369199,-1.12115139781563,
0.9));
#10441=CARTESIAN_POINT('Ctrl Pts',(11.6765943959699,-1.38252448313292,0.9));
#10442=CARTESIAN_POINT('Ctrl Pts',(10.0577014803155,-1.54155822929668,0.900004386952174));
#10443=CARTESIAN_POINT('Ctrl Pts',(7.35045927226653,-1.74750661992774,0.90000020513805));
#10444=CARTESIAN_POINT('Ctrl Pts',(3.54497585078588,-1.67885197560093,0.899998846478116));
#10445=CARTESIAN_POINT('Ctrl Pts',(1.38372480803625,-1.41002339692611,0.900007381454799));
#10446=CARTESIAN_POINT('Ctrl Pts',(0.315675209020016,-1.2059043252356,0.9));
#10447=CARTESIAN_POINT('Ctrl Pts',(11.6912432102654,-1.53175516862908,0.830242007927396));
#10448=CARTESIAN_POINT('Ctrl Pts',(10.070172518288,-1.69119563674726,0.830042231904815));
#10449=CARTESIAN_POINT('Ctrl Pts',(7.35645297288469,-1.89806162871739,0.829725685238203));
#10450=CARTESIAN_POINT('Ctrl Pts',(3.53503777381493,-1.8291593714544,0.829829026055289));
#10451=CARTESIAN_POINT('Ctrl Pts',(1.36192166831068,-1.55847530615989,0.830279056498203));
#10452=CARTESIAN_POINT('Ctrl Pts',(0.28762358730286,-1.35283178372728,0.830616544072481));
#10453=CARTESIAN_POINT('Ctrl Pts',(11.6970428895979,-1.59083777456472,0.681858145263203));
#10454=CARTESIAN_POINT('Ctrl Pts',(10.0750816081461,-1.75021732245097,0.681339641080976));
#10455=CARTESIAN_POINT('Ctrl Pts',(7.3588078744758,-1.95708146899443,0.680519979048775));
#10456=CARTESIAN_POINT('Ctrl Pts',(3.53113644431293,-1.88819699008302,0.68078748362792));
#10457=CARTESIAN_POINT('Ctrl Pts',(1.35331700817769,-1.61730376958615,0.681953432622034));
#10458=CARTESIAN_POINT('Ctrl Pts',(0.276437927844241,-1.41141950219787,
0.682830994206899));
#10459=CARTESIAN_POINT('Ctrl Pts',(11.6974038588243,-1.59451504727786,0.617085749108931));
#10460=CARTESIAN_POINT('Ctrl Pts',(10.0753786444688,-1.75377172884558,0.616473434532366));
#10461=CARTESIAN_POINT('Ctrl Pts',(7.35893161235257,-1.96044797105896,0.61550283428964));
#10462=CARTESIAN_POINT('Ctrl Pts',(3.53092277948893,-1.89162724517065,0.615818637525046));
#10463=CARTESIAN_POINT('Ctrl Pts',(1.35277799022997,-1.62098550016515,0.617200513836093));
#10464=CARTESIAN_POINT('Ctrl Pts',(0.27570015339368,-1.4152837823473,0.618237860411764));
#10465=CARTESIAN_POINT('Ctrl Pts',(0.27570015339368,-1.4152837823473,0.618237860411764));
#10466=CARTESIAN_POINT('Ctrl Pts',(1.35277799022997,-1.62098550016515,0.617200513836093));
#10467=CARTESIAN_POINT('Ctrl Pts',(3.53092277948893,-1.89162724517065,0.615818637525046));
#10468=CARTESIAN_POINT('Ctrl Pts',(7.35893161235257,-1.96044797105896,0.61550283428964));
#10469=CARTESIAN_POINT('Ctrl Pts',(10.0753786444688,-1.75377172884558,0.616473434532366));
#10470=CARTESIAN_POINT('Ctrl Pts',(11.6974038588243,-1.59451504727786,0.617085749108931));
#10471=CARTESIAN_POINT('Ctrl Pts',(11.6681436286308,-1.2964346619681,0.9));
#10472=CARTESIAN_POINT('Ctrl Pts',(10.0505146497799,-1.45522470190849,0.9));
#10473=CARTESIAN_POINT('Ctrl Pts',(7.34698379851713,-1.66064017564263,0.9));
#10474=CARTESIAN_POINT('Ctrl Pts',(3.5507249968367,-1.5921338472202,0.9));
#10475=CARTESIAN_POINT('Ctrl Pts',(1.39628032950236,-1.32437289587156,0.9));
#10476=CARTESIAN_POINT('Ctrl Pts',(0.331856371369199,-1.12115139781563,
0.9));
#10477=CARTESIAN_POINT('Ctrl Pts',(12.0003454972153,-1.32890342861544,-0.00659247958978532));
#10478=CARTESIAN_POINT('Ctrl Pts',(11.9894744951615,-1.31808026232082,0.200838596530835));
#10479=CARTESIAN_POINT('Ctrl Pts',(11.9786034924455,-1.30725733885828,0.408269685287046));
#10480=CARTESIAN_POINT('Ctrl Pts',(11.9677324890572,-1.2964346619681,0.615700786872884));
#10481=CARTESIAN_POINT('Ctrl Pts',(12.000116620981,-1.41283311850955,-0.00222526087931226));
#10482=CARTESIAN_POINT('Ctrl Pts',(11.9892453109784,-1.40200002127642,0.205205215027088));
#10483=CARTESIAN_POINT('Ctrl Pts',(11.9783750177566,-1.39116761830557,0.412635780645844));
#10484=CARTESIAN_POINT('Ctrl Pts',(11.9675037034976,-1.38033490526933,0.620066275407343));
#10485=CARTESIAN_POINT('Ctrl Pts',(11.9341774721098,-1.5584705948029,0.00191796595980313));
#10486=CARTESIAN_POINT('Ctrl Pts',(11.9233226835938,-1.54762133657986,0.209348350794306));
#10487=CARTESIAN_POINT('Ctrl Pts',(11.9124678718222,-1.53677206634062,0.416778732304926));
#10488=CARTESIAN_POINT('Ctrl Pts',(11.9016132473252,-1.52592301942363,0.624209134118803));
#10489=CARTESIAN_POINT('Ctrl Pts',(11.7925116537096,-1.62071287545028,-0.0022587989925734));
#10490=CARTESIAN_POINT('Ctrl Pts',(11.7816834491585,-1.6098745265243,0.205173499361722));
#10491=CARTESIAN_POINT('Ctrl Pts',(11.7708551999607,-1.59903658749835,0.41260581547062));
#10492=CARTESIAN_POINT('Ctrl Pts',(11.760027440985,-1.58819854843564,0.620038149897102));
#10493=CARTESIAN_POINT('Ctrl Pts',(11.7298629188572,-1.62699926142283,-0.0052140742384003));
#10494=CARTESIAN_POINT('Ctrl Pts',(11.7190429637906,-1.61617098622686,0.202219177289036));
#10495=CARTESIAN_POINT('Ctrl Pts',(11.708223275703,-1.60534291388117,0.409652451626141));
#10496=CARTESIAN_POINT('Ctrl Pts',(11.6974038588243,-1.59451504727786,0.617085749108931));
#10497=CARTESIAN_POINT('Ctrl Pts',(12.,-1.32855945177638,-1.94722710178397E-16));
#10498=CARTESIAN_POINT('Ctrl Pts',(11.9892441636707,-1.31785094954632,0.205233583190348));
#10499=CARTESIAN_POINT('Ctrl Pts',(11.978488326693,-1.30714268506935,0.410467178751997));
#10500=CARTESIAN_POINT('Ctrl Pts',(11.9677324890572,-1.2964346619681,0.615700786872884));
#10501=CARTESIAN_POINT('Ctrl Pts',(11.6974038588243,-1.59451504727786,0.617085749108931));
#10502=CARTESIAN_POINT('Ctrl Pts',(11.7081326228587,-1.605252190239,0.41139047675572));
#10503=CARTESIAN_POINT('Ctrl Pts',(11.7188616535763,-1.61598953550924,0.205695227161956));
#10504=CARTESIAN_POINT('Ctrl Pts',(11.7295909468525,-1.62672708026858,8.73866951023317E-17));
#10505=CARTESIAN_POINT('Ctrl Pts',(11.7298546566854,1.62699099289774,-0.00505567716946009));
#10506=CARTESIAN_POINT('Ctrl Pts',(11.719037455812,1.61616547398006,0.202324775346606));
#10507=CARTESIAN_POINT('Ctrl Pts',(11.7082205217827,1.60534015781013,0.409705250660816));
#10508=CARTESIAN_POINT('Ctrl Pts',(11.6974038588243,1.59451504727786,0.617085749108931));
#10509=CARTESIAN_POINT('Ctrl Pts',(11.8133862946664,1.61860913476435,-0.00111531114554236));
#10510=CARTESIAN_POINT('Ctrl Pts',(11.8025579038448,1.6077699189899,0.206263846261978));
#10511=CARTESIAN_POINT('Ctrl Pts',(11.7917299466398,1.59693199028804,0.41364309356145));
#10512=CARTESIAN_POINT('Ctrl Pts',(11.7809019683719,1.58609304882157,0.621022283493159));
#10513=CARTESIAN_POINT('Ctrl Pts',(11.9519653779615,1.53884931758497,0.00198566945999789));
#10514=CARTESIAN_POINT('Ctrl Pts',(11.9411087765487,1.52800449744246,0.209363119024413));
#10515=CARTESIAN_POINT('Ctrl Pts',(11.9302521502216,1.51715965702667,0.416740564833343));
#10516=CARTESIAN_POINT('Ctrl Pts',(11.9193956662674,1.50631506689811,0.624118030142866));
#10517=CARTESIAN_POINT('Ctrl Pts',(12.0001655389052,1.39184242582033,-0.00315867047762133));
#10518=CARTESIAN_POINT('Ctrl Pts',(11.9892972278067,1.38101476165208,0.204219175612729));
#10519=CARTESIAN_POINT('Ctrl Pts',(11.9784292129672,1.37018709651964,0.41159703650799));
#10520=CARTESIAN_POINT('Ctrl Pts',(11.9675608998875,1.35935984444403,0.618974903273729));
#10521=CARTESIAN_POINT('Ctrl Pts',(12.0003371960637,1.32889516399154,-0.00643408418199817));
#10522=CARTESIAN_POINT('Ctrl Pts',(11.9894689610601,1.31807475269516,0.200944193475792));
#10523=CARTESIAN_POINT('Ctrl Pts',(11.9786007253947,1.3072545841082,0.408322483762789));
#10524=CARTESIAN_POINT('Ctrl Pts',(11.9677324890572,1.2964346619681,0.615700786872884));
#10525=CARTESIAN_POINT('Ctrl Pts',(11.7295909468525,1.62672708026857,-8.50014503228635E-17));
#10526=CARTESIAN_POINT('Ctrl Pts',(11.7188616535763,1.61598953550924,0.205695227161956));
#10527=CARTESIAN_POINT('Ctrl Pts',(11.7081326228587,1.605252190239,0.411390476755719));
#10528=CARTESIAN_POINT('Ctrl Pts',(11.6974038588243,1.59451504727786,0.617085749108931));
#10529=CARTESIAN_POINT('Ctrl Pts',(11.9677324890572,1.2964346619681,0.615700786872884));
#10530=CARTESIAN_POINT('Ctrl Pts',(11.978488326693,1.30714268506935,0.410467178751997));
#10531=CARTESIAN_POINT('Ctrl Pts',(11.9892441636707,1.31785094954633,0.205233583190349));
#10532=CARTESIAN_POINT('Ctrl Pts',(12.,1.32855945177638,-2.38524477946811E-17));
#10533=CARTESIAN_POINT('Ctrl Pts',(0.3318563713692,1.12115139781563,0.9));
#10534=CARTESIAN_POINT('Ctrl Pts',(1.92849230856897,1.42598364489954,0.9));
#10535=CARTESIAN_POINT('Ctrl Pts',(5.71993880054687,1.76935652211139,0.9));
#10536=CARTESIAN_POINT('Ctrl Pts',(9.51130499016288,1.50815471522196,0.9));
#10537=CARTESIAN_POINT('Ctrl Pts',(11.6681436286308,1.2964346619681,0.9));
#10538=CARTESIAN_POINT('Ctrl Pts',(0.315675209020018,1.2059043252356,0.9));
#10539=CARTESIAN_POINT('Ctrl Pts',(1.91774960754439,1.51208293277137,0.900011072182198));
#10540=CARTESIAN_POINT('Ctrl Pts',(5.72069615836457,1.85663493780214,0.899990666655967));
#10541=CARTESIAN_POINT('Ctrl Pts',(9.5180705084307,1.59456947801794,0.900005849269565));
#10542=CARTESIAN_POINT('Ctrl Pts',(11.6765943959699,1.38252448313292,0.9));
#10543=CARTESIAN_POINT('Ctrl Pts',(0.287623587302861,1.35283178372728,0.83061654407248));
#10544=CARTESIAN_POINT('Ctrl Pts',(1.89907070881462,1.6612970673762,0.830110312711064));
#10545=CARTESIAN_POINT('Ctrl Pts',(5.72203120258494,2.00791989451774,0.829536565111056));
#10546=CARTESIAN_POINT('Ctrl Pts',(9.52981562096212,1.74434245945332,0.829975639897288));
#10547=CARTESIAN_POINT('Ctrl Pts',(11.6912432102654,1.53175516862908,0.830242007927395));
#10548=CARTESIAN_POINT('Ctrl Pts',(0.276437927844243,1.41141950219787,0.682830994206899));
#10549=CARTESIAN_POINT('Ctrl Pts',(1.89175654834445,1.7202459032803,0.681514651829601));
#10550=CARTESIAN_POINT('Ctrl Pts',(5.72254254462207,2.06699613896002,0.680031275065471));
#10551=CARTESIAN_POINT('Ctrl Pts',(9.53442784766217,1.80334383841306,0.681166806353567));
#10552=CARTESIAN_POINT('Ctrl Pts',(11.6970428895979,1.59083777456472,0.681858145263204));
#10553=CARTESIAN_POINT('Ctrl Pts',(0.275700153393682,1.4152837823473,0.618237860411764));
#10554=CARTESIAN_POINT('Ctrl Pts',(1.89131690864814,1.72383635907408,0.616681840548257));
#10555=CARTESIAN_POINT('Ctrl Pts',(5.72257555688819,2.07025489722917,0.614922376024419));
#10556=CARTESIAN_POINT('Ctrl Pts',(9.53470357301702,1.80685728936816,0.616269329673511));
#10557=CARTESIAN_POINT('Ctrl Pts',(11.6974038588243,1.59451504727786,0.617085749108931));
#10558=CARTESIAN_POINT('Ctrl Pts',(11.6974038588243,1.59451504727786,0.617085749108931));
#10559=CARTESIAN_POINT('Ctrl Pts',(9.53470357301702,1.80685728936816,0.616269329673511));
#10560=CARTESIAN_POINT('Ctrl Pts',(5.72257555688819,2.07025489722917,0.614922376024419));
#10561=CARTESIAN_POINT('Ctrl Pts',(1.89131690864814,1.72383635907408,0.616681840548257));
#10562=CARTESIAN_POINT('Ctrl Pts',(0.275700153393682,1.4152837823473,0.618237860411764));
#10563=CARTESIAN_POINT('Ctrl Pts',(0.3318563713692,1.12115139781563,0.9));
#10564=CARTESIAN_POINT('Ctrl Pts',(1.92849230856897,1.42598364489954,0.9));
#10565=CARTESIAN_POINT('Ctrl Pts',(5.71993880054687,1.76935652211139,0.9));
#10566=CARTESIAN_POINT('Ctrl Pts',(9.51130499016288,1.50815471522196,0.9));
#10567=CARTESIAN_POINT('Ctrl Pts',(11.6681436286308,1.2964346619681,0.9));
#10568=CARTESIAN_POINT('Ctrl Pts',(-0.000343174493958709,1.15350944952984,
-0.00654815942696785));
#10569=CARTESIAN_POINT('Ctrl Pts',(0.0105270529019337,1.14272303380391,
0.200868135340743));
#10570=CARTESIAN_POINT('Ctrl Pts',(0.0213972813757523,1.13193701467556,
0.408284450676511));
#10571=CARTESIAN_POINT('Ctrl Pts',(0.0322675109428289,1.12115139781563,
0.615700786872884));
#10572=CARTESIAN_POINT('Ctrl Pts',(-0.000129060241737355,1.23228777111366,
-0.0024626161135415));
#10573=CARTESIAN_POINT('Ctrl Pts',(0.0107416412387167,1.22148297235423,
0.204952596860618));
#10574=CARTESIAN_POINT('Ctrl Pts',(0.0216107531875107,1.21067920461451,
0.412367946918899));
#10575=CARTESIAN_POINT('Ctrl Pts',(0.0324814606290031,1.19987501734845,
0.61978319007907));
#10576=CARTESIAN_POINT('Ctrl Pts',(0.0574602827844584,1.36931747586956,
0.00164530659801973));
#10577=CARTESIAN_POINT('Ctrl Pts',(0.0683025556324749,1.35848226928888,
0.209060253413207));
#10578=CARTESIAN_POINT('Ctrl Pts',(0.079145272670006,1.34764679267913,0.416475160658282));
#10579=CARTESIAN_POINT('Ctrl Pts',(0.0899872847341513,1.33681188280878,
0.62389013300849));
#10580=CARTESIAN_POINT('Ctrl Pts',(0.185325846363896,1.43651931939441,-0.00156109881554352));
#10581=CARTESIAN_POINT('Ctrl Pts',(0.196119220517603,1.4256988926218,0.205857093047737));
#10582=CARTESIAN_POINT('Ctrl Pts',(0.20691256009293,1.41487906031557,0.413275315721495));
#10583=CARTESIAN_POINT('Ctrl Pts',(0.217705180746507,1.40405902353128,0.620693562444772));
#10584=CARTESIAN_POINT('Ctrl Pts',(0.243371723604776,1.44769625339383,-0.00402191236404));
#10585=CARTESIAN_POINT('Ctrl Pts',(0.254148334883323,1.43689183478419,0.203397976373256));
#10586=CARTESIAN_POINT('Ctrl Pts',(0.264924480472538,1.42608767680315,0.410817900476086));
#10587=CARTESIAN_POINT('Ctrl Pts',(0.275700153393682,1.4152837823473,0.618237860411764));
#10588=CARTESIAN_POINT('Ctrl Pts',(-1.23734572934908E-17,1.15316892111333,
-8.67361737988404E-19));
#10589=CARTESIAN_POINT('Ctrl Pts',(0.0107558359204753,1.14249602316336,
0.205233575389367));
#10590=CARTESIAN_POINT('Ctrl Pts',(0.0215116728964674,1.13182351356624,
0.410467170919192));
#10591=CARTESIAN_POINT('Ctrl Pts',(0.0322675109428289,1.12115139781563,
0.615700786872884));
#10592=CARTESIAN_POINT('Ctrl Pts',(0.275700153393682,1.4152837823473,0.618237860411764));
#10593=CARTESIAN_POINT('Ctrl Pts',(0.264994127943615,1.42601784692504,0.412158538389472));
#10594=CARTESIAN_POINT('Ctrl Pts',(0.254287635915814,1.43675217163244,0.206079251738322));
#10595=CARTESIAN_POINT('Ctrl Pts',(0.243580684154575,1.44748675362873,-1.9298798670242E-17));
#10596=CARTESIAN_POINT('Ctrl Pts',(11.7295909468525,-1.62672708026858,0.));
#10597=CARTESIAN_POINT('Ctrl Pts',(11.7192775324813,-1.61592692249094,0.206079286804135));
#10598=CARTESIAN_POINT('Ctrl Pts',(11.70896411811,-1.6051267647133,0.41215857360827));
#10599=CARTESIAN_POINT('Ctrl Pts',(11.6986507037388,-1.59432660693566,0.618237860412405));
#10600=CARTESIAN_POINT('Ctrl Pts',(7.90092085928651,-2.00057770191527,0.));
#10601=CARTESIAN_POINT('Ctrl Pts',(7.89749915175266,-1.98977754413763,0.206079286804135));
#10602=CARTESIAN_POINT('Ctrl Pts',(7.89407744421881,-1.97897738636,0.41215857360827));
#10603=CARTESIAN_POINT('Ctrl Pts',(7.89065573668496,-1.96817722858236,0.618237860412405));
#10604=CARTESIAN_POINT('Ctrl Pts',(4.07225077172054,-2.17467835246083,0.));
#10605=CARTESIAN_POINT('Ctrl Pts',(4.07572077102407,-2.16387819468319,0.206079286804135));
#10606=CARTESIAN_POINT('Ctrl Pts',(4.07919077032759,-2.15307803690555,0.41215857360827));
#10607=CARTESIAN_POINT('Ctrl Pts',(4.08266076963111,-2.14227787912792,0.618237860412405));
#10608=CARTESIAN_POINT('Ctrl Pts',(0.243580684154574,-1.44748675362873,
0.));
#10609=CARTESIAN_POINT('Ctrl Pts',(0.253942390295469,-1.43668659585109,
0.206079286804135));
#10610=CARTESIAN_POINT('Ctrl Pts',(0.264304096436365,-1.42588643807345,
0.41215857360827));
#10611=CARTESIAN_POINT('Ctrl Pts',(0.27466580257726,-1.41508628029581,0.618237860412405));
#10612=CARTESIAN_POINT('Origin',(0.,-1.4,0.));
#10613=CARTESIAN_POINT('Origin',(6.08012166120517,1.06803409199199E-16,
0.9));
#10614=CARTESIAN_POINT('Ctrl Pts',(0.243580684154574,1.44748675362873,0.));
#10615=CARTESIAN_POINT('Ctrl Pts',(0.253942390295469,1.43668659585109,0.206079286804135));
#10616=CARTESIAN_POINT('Ctrl Pts',(0.264304096436365,1.42588643807345,0.41215857360827));
#10617=CARTESIAN_POINT('Ctrl Pts',(0.27466580257726,1.41508628029581,0.618237860412405));
#10618=CARTESIAN_POINT('Ctrl Pts',(4.07225077172054,2.17467835246083,0.));
#10619=CARTESIAN_POINT('Ctrl Pts',(4.07572077102407,2.16387819468319,0.206079286804135));
#10620=CARTESIAN_POINT('Ctrl Pts',(4.07919077032759,2.15307803690555,0.41215857360827));
#10621=CARTESIAN_POINT('Ctrl Pts',(4.08266076963111,2.14227787912792,0.618237860412405));
#10622=CARTESIAN_POINT('Ctrl Pts',(7.90092085928651,2.00057770191527,0.));
#10623=CARTESIAN_POINT('Ctrl Pts',(7.89749915175266,1.98977754413763,0.206079286804135));
#10624=CARTESIAN_POINT('Ctrl Pts',(7.89407744421881,1.97897738636,0.41215857360827));
#10625=CARTESIAN_POINT('Ctrl Pts',(7.89065573668496,1.96817722858236,0.618237860412405));
#10626=CARTESIAN_POINT('Ctrl Pts',(11.7295909468525,1.62672708026858,0.));
#10627=CARTESIAN_POINT('Ctrl Pts',(11.7192775324813,1.61592692249094,0.206079286804135));
#10628=CARTESIAN_POINT('Ctrl Pts',(11.70896411811,1.6051267647133,0.41215857360827));
#10629=CARTESIAN_POINT('Ctrl Pts',(11.6986507037388,1.59432660693566,0.618237860412405));
#10630=CARTESIAN_POINT('Origin',(12.,1.6,0.));
#18335=UNCERTAINTY_MEASURE_WITH_UNIT(LENGTH_MEASURE(0.001),#18354,
'DISTANCE_ACCURACY_VALUE',
'Maximum model space distance between geometric entities at asserted c
onnectivities');
#18341=UNCERTAINTY_MEASURE_WITH_UNIT(LENGTH_MEASURE(0.001),#18354,
'DISTANCE_ACCURACY_VALUE',
'Maximum model space distance between geometric entities at asserted c
onnectivities');
#18347=(
GEOMETRIC_REPRESENTATION_CONTEXT(3)
GLOBAL_UNCERTAINTY_ASSIGNED_CONTEXT((#18335))
GLOBAL_UNIT_ASSIGNED_CONTEXT((#18354,#18356,#18357))
REPRESENTATION_CONTEXT('','3D')
);
#18353=(
GEOMETRIC_REPRESENTATION_CONTEXT(3)
GLOBAL_UNCERTAINTY_ASSIGNED_CONTEXT((#18341))
GLOBAL_UNIT_ASSIGNED_CONTEXT((#18354,#18356,#18357))
REPRESENTATION_CONTEXT('','3D')
);
#18354=(
LENGTH_UNIT()
NAMED_UNIT(*)
SI_UNIT(.CENTI.,.METRE.)
);
#18356=(
NAMED_UNIT(*)
PLANE_ANGLE_UNIT()
SI_UNIT($,.RADIAN.)
);
#18357=(
NAMED_UNIT(*)
SI_UNIT($,.STERADIAN.)
SOLID_ANGLE_UNIT()
);
#18363=SHAPE_DEFINITION_REPRESENTATION(#18374,#18401);
#18374=PRODUCT_DEFINITION_SHAPE('',$,#18413);
#18401=SHAPE_REPRESENTATION('',(#6686),#18347);
#18407=PRODUCT_DEFINITION_CONTEXT('part definition',#18442,'design');
#18413=PRODUCT_DEFINITION('2026-11-10-01-32-12-355',
'Upper structural shell',#18424,#18407);
#18424=PRODUCT_DEFINITION_FORMATION('',$,#18449);
#18442=APPLICATION_CONTEXT(
'Core Data for Automotive Mechanical Design Process');
#18443=PRODUCT_CONTEXT('part definition',#18442,'mechanical');
#18449=PRODUCT('2026-11-10-01-32-12-355','Upper structural shell',$,(#18443));
#18459=PRESENTATION_STYLE_ASSIGNMENT((#18467));
#18467=SURFACE_STYLE_USAGE(.BOTH.,#18475);
#18475=SURFACE_SIDE_STYLE('',(#18483));
#18483=SURFACE_STYLE_FILL_AREA(#18491);
#18491=FILL_AREA_STYLE('Structural dark blue',(#18499));
#18499=FILL_AREA_STYLE_COLOUR('Structural dark blue',#18507);
#18507=COLOUR_RGB('Structural dark blue',0.0901960784313725,0.270588235294118,
0.513725490196078);
ENDSEC;
END-ISO-10303-21;
